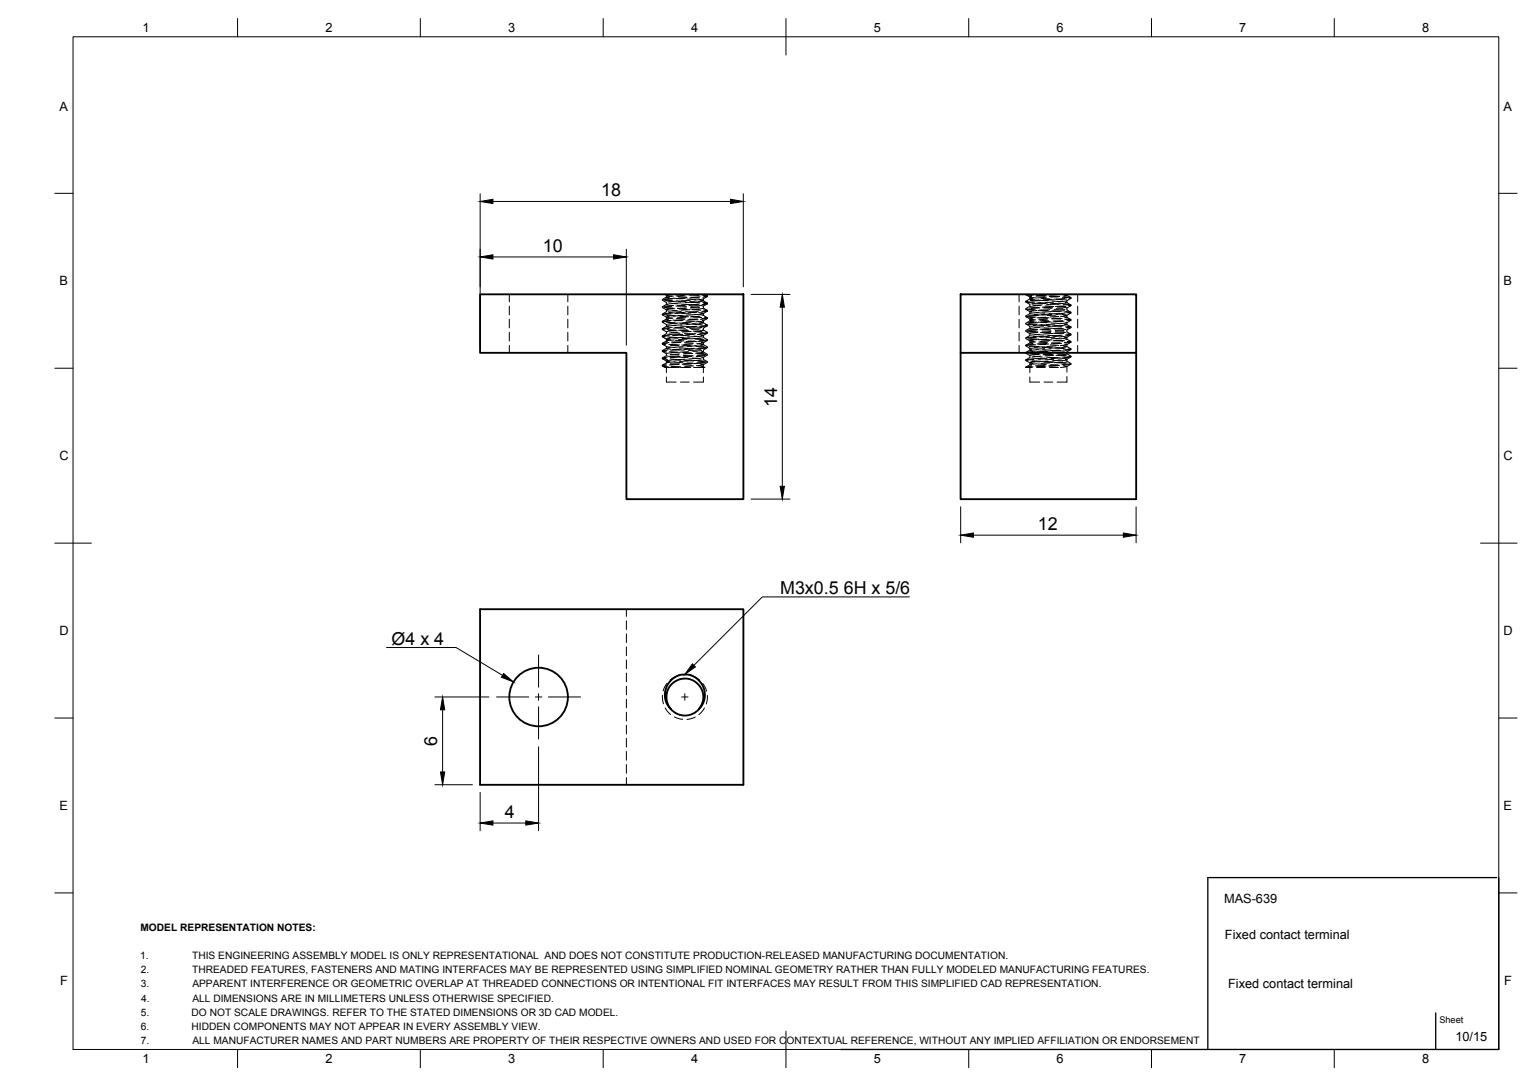
ISO-10303-21;
HEADER;
/* Generated by software containing ST-Developer
 * from STEP Tools, Inc. (www.steptools.com) 
 */

FILE_DESCRIPTION(
/* description */ ('Independent maintained push-to-latch/pull-to-reset mushroom-operator 
CAD. Two opposed spring-loaded ball detents in turned circular seats b
ias both travel stops; direct normally-closed bridge opens6mm when pre
ssed. Rounded palm/pull rim, captured head screw, removable detent clo
sures, native Coil spring families, insulated shared terminals and ord
inary machining features. Manual geometric states and ideal same-mater
ial spring-energy direction only; no electrical/safety certification, 
force/contact dynamics, wear, load or life rating. Requested blue/gray
 visual palette, not safety identification. External wiring/anchors an
d application engineering omitted.'),
/* implementation_level */ '2;1');

FILE_NAME(
/* name */ 'Fixed contact terminal.step',
/* time_stamp */ '2026-11-08T17:54:26-08:00',
/* author */ (''),
/* organization */ (''),
/* preprocessor_version */ 'ST-DEVELOPER v20.2',
/* originating_system */ 'Autodesk Translation Framework v15.17.0.0',
/* authorisation */ '');

FILE_SCHEMA (('AUTOMOTIVE_DESIGN { 1 0 10303 214 3 1 1 }'));
ENDSEC;

DATA;
#10=MECHANICAL_DESIGN_GEOMETRIC_PRESENTATION_REPRESENTATION('',(#198),#43980);
#164=SHAPE_REPRESENTATION_RELATIONSHIP('SRR','None',#44064,#181);
#181=ADVANCED_BREP_SHAPE_REPRESENTATION('',(#215),#43971);
#198=STYLED_ITEM('',(#44154),#215);
#215=MANIFOLD_SOLID_BREP('Body1',#11239);
#247=B_SPLINE_SURFACE_WITH_KNOTS('',3,3,((#35123,#35124,#35125,#35126,#35127,
#35128,#35129,#35130,#35131,#35132,#35133,#35134,#35135,#35136,#35137,#35138,
#35139,#35140,#35141,#35142,#35143,#35144,#35145,#35146,#35147,#35148,#35149,
#35150,#35151,#35152,#35153,#35154,#35155,#35156,#35157,#35158,#35159,#35160,
#35161,#35162,#35163,#35164,#35165,#35166,#35167,#35168,#35169,#35170,#35171,
#35172,#35173,#35174,#35175,#35176,#35177,#35178,#35179,#35180,#35181,#35182,
#35183,#35184,#35185,#35186,#35187,#35188,#35189,#35190),(#35191,#35192,
#35193,#35194,#35195,#35196,#35197,#35198,#35199,#35200,#35201,#35202,#35203,
#35204,#35205,#35206,#35207,#35208,#35209,#35210,#35211,#35212,#35213,#35214,
#35215,#35216,#35217,#35218,#35219,#35220,#35221,#35222,#35223,#35224,#35225,
#35226,#35227,#35228,#35229,#35230,#35231,#35232,#35233,#35234,#35235,#35236,
#35237,#35238,#35239,#35240,#35241,#35242,#35243,#35244,#35245,#35246,#35247,
#35248,#35249,#35250,#35251,#35252,#35253,#35254,#35255,#35256,#35257,#35258),
(#35259,#35260,#35261,#35262,#35263,#35264,#35265,#35266,#35267,#35268,
#35269,#35270,#35271,#35272,#35273,#35274,#35275,#35276,#35277,#35278,#35279,
#35280,#35281,#35282,#35283,#35284,#35285,#35286,#35287,#35288,#35289,#35290,
#35291,#35292,#35293,#35294,#35295,#35296,#35297,#35298,#35299,#35300,#35301,
#35302,#35303,#35304,#35305,#35306,#35307,#35308,#35309,#35310,#35311,#35312,
#35313,#35314,#35315,#35316,#35317,#35318,#35319,#35320,#35321,#35322,#35323,
#35324,#35325,#35326),(#35327,#35328,#35329,#35330,#35331,#35332,#35333,
#35334,#35335,#35336,#35337,#35338,#35339,#35340,#35341,#35342,#35343,#35344,
#35345,#35346,#35347,#35348,#35349,#35350,#35351,#35352,#35353,#35354,#35355,
#35356,#35357,#35358,#35359,#35360,#35361,#35362,#35363,#35364,#35365,#35366,
#35367,#35368,#35369,#35370,#35371,#35372,#35373,#35374,#35375,#35376,#35377,
#35378,#35379,#35380,#35381,#35382,#35383,#35384,#35385,#35386,#35387,#35388,
#35389,#35390,#35391,#35392,#35393,#35394)),.UNSPECIFIED.,.F.,.F.,.F.,(4,
4),(4,1,1,1,1,1,1,1,1,1,1,1,1,1,1,1,1,1,1,1,1,1,1,1,1,1,1,1,1,1,1,1,1,1,
1,1,1,1,1,1,1,1,1,1,1,1,1,1,1,1,1,1,1,1,1,1,1,1,1,1,1,1,1,1,1,4),(0.,0.0321584099938621),
(11.8553612635792,12.8530908876339,13.8508205116886,14.8485501357432,15.8462797597979,
16.8440093838525,17.8417390079072,18.8394686319618,19.8371982560165,20.8349278800712,
21.8326575041258,22.8303871281805,23.8281167522351,24.8258463762898,25.8235760003445,
26.8213056243991,27.8190352484538,28.8167648725084,29.8144944965631,30.8122241206177,
31.8099537446724,32.8076833687271,33.8054129927817,34.8031426168364,35.800872240891,
36.7986018649457,37.7963314890004,38.794061113055,39.7917907371097,40.7895203611643,
41.787249985219,42.7849796092736,43.7827092333283,44.780438857383,45.7781684814376,
46.7758981054923,47.7736277295469,48.7713573536016,49.7690869776563,50.7668166017109,
51.7645462257656,52.7622758498202,53.7600054738749,54.7577350979295,55.7554647219842,
56.7531943460389,57.7509239700935,58.7486535941482,59.7463832182028,60.7441128422575,
61.7418424663121,62.7395720903668,63.7373017144215,64.7350313384761,65.7327609625308,
66.7304905865854,67.7282202106401,68.7259498346948,69.7236794587494,70.7214090828041,
71.7191387068587,72.7168683309134,73.7145979549681,74.7123275790227,75.7100572030774,
76.707786827132),.UNSPECIFIED.);
#248=B_SPLINE_SURFACE_WITH_KNOTS('',3,3,((#35469,#35470,#35471,#35472,#35473,
#35474,#35475,#35476,#35477,#35478,#35479,#35480,#35481,#35482,#35483,#35484,
#35485,#35486,#35487,#35488,#35489,#35490,#35491,#35492,#35493,#35494,#35495,
#35496,#35497,#35498,#35499,#35500,#35501,#35502,#35503,#35504,#35505,#35506,
#35507,#35508,#35509,#35510,#35511,#35512,#35513,#35514,#35515,#35516,#35517,
#35518,#35519,#35520,#35521,#35522,#35523,#35524,#35525,#35526,#35527,#35528,
#35529,#35530,#35531,#35532,#35533,#35534,#35535,#35536),(#35537,#35538,
#35539,#35540,#35541,#35542,#35543,#35544,#35545,#35546,#35547,#35548,#35549,
#35550,#35551,#35552,#35553,#35554,#35555,#35556,#35557,#35558,#35559,#35560,
#35561,#35562,#35563,#35564,#35565,#35566,#35567,#35568,#35569,#35570,#35571,
#35572,#35573,#35574,#35575,#35576,#35577,#35578,#35579,#35580,#35581,#35582,
#35583,#35584,#35585,#35586,#35587,#35588,#35589,#35590,#35591,#35592,#35593,
#35594,#35595,#35596,#35597,#35598,#35599,#35600,#35601,#35602,#35603,#35604),
(#35605,#35606,#35607,#35608,#35609,#35610,#35611,#35612,#35613,#35614,
#35615,#35616,#35617,#35618,#35619,#35620,#35621,#35622,#35623,#35624,#35625,
#35626,#35627,#35628,#35629,#35630,#35631,#35632,#35633,#35634,#35635,#35636,
#35637,#35638,#35639,#35640,#35641,#35642,#35643,#35644,#35645,#35646,#35647,
#35648,#35649,#35650,#35651,#35652,#35653,#35654,#35655,#35656,#35657,#35658,
#35659,#35660,#35661,#35662,#35663,#35664,#35665,#35666,#35667,#35668,#35669,
#35670,#35671,#35672),(#35673,#35674,#35675,#35676,#35677,#35678,#35679,
#35680,#35681,#35682,#35683,#35684,#35685,#35686,#35687,#35688,#35689,#35690,
#35691,#35692,#35693,#35694,#35695,#35696,#35697,#35698,#35699,#35700,#35701,
#35702,#35703,#35704,#35705,#35706,#35707,#35708,#35709,#35710,#35711,#35712,
#35713,#35714,#35715,#35716,#35717,#35718,#35719,#35720,#35721,#35722,#35723,
#35724,#35725,#35726,#35727,#35728,#35729,#35730,#35731,#35732,#35733,#35734,
#35735,#35736,#35737,#35738,#35739,#35740)),.UNSPECIFIED.,.F.,.F.,.F.,(4,
4),(4,1,1,1,1,1,1,1,1,1,1,1,1,1,1,1,1,1,1,1,1,1,1,1,1,1,1,1,1,1,1,1,1,1,
1,1,1,1,1,1,1,1,1,1,1,1,1,1,1,1,1,1,1,1,1,1,1,1,1,1,1,1,1,1,1,4),(0.,0.0321584099938616),
(14.3984001269718,15.3961297510265,16.3938593750811,17.3915889991358,18.3893186231905,
19.3870482472451,20.3847778712998,21.3825074953544,22.3802371194091,23.3779667434637,
24.3756963675184,25.3734259915731,26.3711556156277,27.3688852396824,28.366614863737,
29.3643444877917,30.3620741118463,31.359803735901,32.3575333599556,33.3552629840103,
34.352992608065,35.3507222321196,36.3484518561743,37.3461814802289,38.3439111042836,
39.3416407283382,40.3393703523929,41.3370999764475,42.3348296005022,43.3325592245569,
44.3302888486115,45.3280184726662,46.3257480967208,47.3234777207755,48.3212073448301,
49.3189369688848,50.3166665929395,51.3143962169941,52.3121258410488,53.3098554651034,
54.3075850891581,55.3053147132127,56.3030443372674,57.3007739613221,58.2985035853767,
59.2962332094314,60.293962833486,61.2916924575407,62.2894220815953,63.28715170565,
64.2848813297046,65.2826109537593,66.280340577814,67.2780702018686,68.2757998259233,
69.2735294499779,70.2712590740326,71.2689886980872,72.2667183221419,73.2644479461966,
74.2621775702512,75.2599071943059,76.2576368183605,77.2553664424152,78.2530960664698,
79.2508256905245),.UNSPECIFIED.);
#317=FACE_BOUND('',#1609,.T.);
#318=FACE_BOUND('',#1615,.T.);
#319=FACE_BOUND('',#1616,.T.);
#423=PLANE('',#12010);
#424=PLANE('',#12013);
#425=PLANE('',#12017);
#426=PLANE('',#12018);
#427=PLANE('',#12019);
#428=PLANE('',#12020);
#429=PLANE('',#12021);
#430=PLANE('',#12022);
#431=PLANE('',#12023);
#432=PLANE('',#12024);
#899=FACE_OUTER_BOUND('',#1580,.T.);
#900=FACE_OUTER_BOUND('',#1581,.T.);
#901=FACE_OUTER_BOUND('',#1582,.T.);
#902=FACE_OUTER_BOUND('',#1583,.T.);
#903=FACE_OUTER_BOUND('',#1584,.T.);
#904=FACE_OUTER_BOUND('',#1585,.T.);
#905=FACE_OUTER_BOUND('',#1586,.T.);
#906=FACE_OUTER_BOUND('',#1587,.T.);
#907=FACE_OUTER_BOUND('',#1588,.T.);
#908=FACE_OUTER_BOUND('',#1589,.T.);
#909=FACE_OUTER_BOUND('',#1590,.T.);
#910=FACE_OUTER_BOUND('',#1591,.T.);
#911=FACE_OUTER_BOUND('',#1592,.T.);
#912=FACE_OUTER_BOUND('',#1593,.T.);
#913=FACE_OUTER_BOUND('',#1594,.T.);
#914=FACE_OUTER_BOUND('',#1595,.T.);
#915=FACE_OUTER_BOUND('',#1596,.T.);
#916=FACE_OUTER_BOUND('',#1597,.T.);
#917=FACE_OUTER_BOUND('',#1598,.T.);
#918=FACE_OUTER_BOUND('',#1599,.T.);
#919=FACE_OUTER_BOUND('',#1600,.T.);
#920=FACE_OUTER_BOUND('',#1601,.T.);
#921=FACE_OUTER_BOUND('',#1602,.T.);
#922=FACE_OUTER_BOUND('',#1603,.T.);
#923=FACE_OUTER_BOUND('',#1604,.T.);
#924=FACE_OUTER_BOUND('',#1605,.T.);
#925=FACE_OUTER_BOUND('',#1606,.T.);
#926=FACE_OUTER_BOUND('',#1607,.T.);
#927=FACE_OUTER_BOUND('',#1608,.T.);
#928=FACE_OUTER_BOUND('',#1610,.T.);
#929=FACE_OUTER_BOUND('',#1611,.T.);
#930=FACE_OUTER_BOUND('',#1612,.T.);
#931=FACE_OUTER_BOUND('',#1613,.T.);
#932=FACE_OUTER_BOUND('',#1614,.T.);
#933=FACE_OUTER_BOUND('',#1617,.T.);
#1580=EDGE_LOOP('',(#9101,#9102,#9103,#9104,#9105,#9106,#9107,#9108));
#1581=EDGE_LOOP('',(#9109,#9110,#9111,#9112));
#1582=EDGE_LOOP('',(#9113,#9114,#9115,#9116));
#1583=EDGE_LOOP('',(#9117,#9118,#9119,#9120));
#1584=EDGE_LOOP('',(#9121,#9122,#9123,#9124));
#1585=EDGE_LOOP('',(#9125,#9126,#9127,#9128));
#1586=EDGE_LOOP('',(#9129,#9130,#9131,#9132));
#1587=EDGE_LOOP('',(#9133,#9134,#9135,#9136));
#1588=EDGE_LOOP('',(#9137,#9138,#9139,#9140));
#1589=EDGE_LOOP('',(#9141,#9142,#9143,#9144));
#1590=EDGE_LOOP('',(#9145,#9146,#9147,#9148));
#1591=EDGE_LOOP('',(#9149,#9150,#9151,#9152));
#1592=EDGE_LOOP('',(#9153,#9154,#9155,#9156));
#1593=EDGE_LOOP('',(#9157,#9158,#9159,#9160));
#1594=EDGE_LOOP('',(#9161,#9162,#9163,#9164));
#1595=EDGE_LOOP('',(#9165,#9166,#9167,#9168));
#1596=EDGE_LOOP('',(#9169,#9170,#9171,#9172));
#1597=EDGE_LOOP('',(#9173,#9174,#9175,#9176));
#1598=EDGE_LOOP('',(#9177,#9178,#9179,#9180));
#1599=EDGE_LOOP('',(#9181,#9182,#9183,#9184));
#1600=EDGE_LOOP('',(#9185,#9186,#9187,#9188,#9189));
#1601=EDGE_LOOP('',(#9190,#9191,#9192,#9193));
#1602=EDGE_LOOP('',(#9194,#9195,#9196,#9197,#9198,#9199,#9200,#9201,#9202,
#9203,#9204,#9205,#9206,#9207,#9208,#9209,#9210,#9211,#9212,#9213,#9214,
#9215,#9216,#9217));
#1603=EDGE_LOOP('',(#9218,#9219,#9220,#9221,#9222,#9223,#9224,#9225,#9226,
#9227,#9228,#9229,#9230,#9231,#9232,#9233,#9234,#9235,#9236,#9237,#9238,
#9239,#9240,#9241));
#1604=EDGE_LOOP('',(#9242,#9243,#9244,#9245));
#1605=EDGE_LOOP('',(#9246));
#1606=EDGE_LOOP('',(#9247,#9248,#9249,#9250));
#1607=EDGE_LOOP('',(#9251,#9252,#9253,#9254));
#1608=EDGE_LOOP('',(#9255,#9256,#9257,#9258));
#1609=EDGE_LOOP('',(#9259));
#1610=EDGE_LOOP('',(#9260,#9261,#9262,#9263,#9264,#9265));
#1611=EDGE_LOOP('',(#9266,#9267,#9268,#9269));
#1612=EDGE_LOOP('',(#9270,#9271,#9272,#9273,#9274,#9275));
#1613=EDGE_LOOP('',(#9276,#9277,#9278,#9279));
#1614=EDGE_LOOP('',(#9280,#9281,#9282,#9283));
#1615=EDGE_LOOP('',(#9284,#9285,#9286,#9287));
#1616=EDGE_LOOP('',(#9288));
#1617=EDGE_LOOP('',(#9289,#9290,#9291,#9292));
#1947=CIRCLE('',#11985,0.12645);
#1948=CIRCLE('',#11986,0.12645);
#1949=CIRCLE('',#11987,0.12645);
#1950=CIRCLE('',#11997,0.12645);
#1951=CIRCLE('',#11999,0.1543);
#1952=CIRCLE('',#12009,0.1543);
#1953=CIRCLE('',#12015,0.2);
#1954=CIRCLE('',#12016,0.2);
#2561=B_SPLINE_CURVE_WITH_KNOTS('',3,(#34297,#34298,#34299,#34300),
 .UNSPECIFIED.,.F.,.F.,(4,4),(64.1414162127729,64.8524255635527),
 .UNSPECIFIED.);
#2562=B_SPLINE_CURVE_WITH_KNOTS('',3,(#34308,#34309,#34310,#34311,#34312,
#34313,#34314,#34315,#34316,#34317),.UNSPECIFIED.,.F.,.F.,(4,3,3,4),(-62.8318530717959,
-61.8592366913888,-60.8615070673342,-60.401269768986),.UNSPECIFIED.);
#2563=B_SPLINE_CURVE_WITH_KNOTS('',3,(#34322,#34323,#34324,#34325,#34326,
#34327,#34328,#34329,#34330,#34331,#34332,#34333,#34334,#34335,#34336,#34337,
#34338,#34339,#34340,#34341,#34342,#34343,#34344,#34345,#34346),
 .UNSPECIFIED.,.F.,.F.,(4,3,3,3,3,3,3,3,4),(57.8582309055934,57.8683181951701,
58.8660478192247,59.8637774432794,60.861507067334,61.8592366913887,62.8569663154434,
63.854695939498,64.1414162127729),.UNSPECIFIED.);
#2564=B_SPLINE_CURVE_WITH_KNOTS('',3,(#34347,#34348,#34349,#34350,#34351,
#34352,#34353,#34354,#34355,#34356,#34357,#34358,#34359,#34360,#34361,#34362,
#34363,#34364,#34365,#34366,#34367,#34368),.UNSPECIFIED.,.F.,.F.,(4,3,3,
3,3,3,3,4),(-60.401269768986,-59.8637774432795,-58.8660478192248,-57.8683181951702,
-56.8705885711155,-55.8728589470609,-54.8751293230062,-54.1180844618064),
 .UNSPECIFIED.);
#2565=B_SPLINE_CURVE_WITH_KNOTS('',3,(#34373,#34374,#34375,#34376,#34377,
#34378,#34379,#34380,#34381,#34382,#34383,#34384,#34385,#34386,#34387,#34388,
#34389,#34390,#34391,#34392,#34393,#34394),.UNSPECIFIED.,.F.,.F.,(4,3,3,
3,3,3,3,4),(51.5750455984138,51.8819404508421,52.8796700748968,53.8773996989514,
54.8751293230061,55.8728589470608,56.8705885711154,57.8582309055934),
 .UNSPECIFIED.);
#2566=B_SPLINE_CURVE_WITH_KNOTS('',3,(#34395,#34396,#34397,#34398,#34399,
#34400,#34401,#34402,#34403,#34404,#34405,#34406,#34407,#34408,#34409,#34410,
#34411,#34412,#34413,#34414,#34415,#34416,#34417,#34418,#34419),
 .UNSPECIFIED.,.F.,.F.,(4,3,3,3,3,3,3,3,4),(-54.1180844618064,-53.8773996989516,
-52.8796700748969,-51.8819404508422,-50.8842108267876,-49.8864812027329,
-48.8887515786783,-47.8910219546236,-47.8348991546268),.UNSPECIFIED.);
#2567=B_SPLINE_CURVE_WITH_KNOTS('',3,(#34424,#34425,#34426,#34427,#34428,
#34429,#34430,#34431,#34432,#34433,#34434,#34435,#34436,#34437,#34438,#34439,
#34440,#34441,#34442,#34443,#34444,#34445),.UNSPECIFIED.,.F.,.F.,(4,3,3,
3,3,3,3,4),(45.2918602912342,45.8955627065142,46.8932923305688,47.8910219546235,
48.8887515786782,49.8864812027328,50.8842108267875,51.5750455984138),
 .UNSPECIFIED.);
#2568=B_SPLINE_CURVE_WITH_KNOTS('',3,(#34446,#34447,#34448,#34449,#34450,
#34451,#34452,#34453,#34454,#34455,#34456,#34457,#34458,#34459,#34460,#34461,
#34462,#34463,#34464,#34465,#34466,#34467),.UNSPECIFIED.,.F.,.F.,(4,3,3,
3,3,3,3,4),(-47.8348991546268,-46.8932923305689,-45.8955627065143,-44.8978330824596,
-43.900103458405,-42.9023738343503,-41.9046442102957,-41.5517138474472),
 .UNSPECIFIED.);
#2569=B_SPLINE_CURVE_WITH_KNOTS('',3,(#34472,#34473,#34474,#34475,#34476,
#34477,#34478,#34479,#34480,#34481,#34482,#34483,#34484,#34485,#34486,#34487,
#34488,#34489,#34490,#34491,#34492,#34493),.UNSPECIFIED.,.F.,.F.,(4,3,3,
3,3,3,3,4),(39.0086749840546,39.9091849621863,40.9069145862409,41.9046442102956,
42.9023738343502,43.9001034584049,44.8978330824595,45.2918602912342),
 .UNSPECIFIED.);
#2570=B_SPLINE_CURVE_WITH_KNOTS('',3,(#34494,#34495,#34496,#34497,#34498,
#34499,#34500,#34501,#34502,#34503,#34504,#34505,#34506,#34507,#34508,#34509,
#34510,#34511,#34512,#34513,#34514,#34515),.UNSPECIFIED.,.F.,.F.,(4,3,3,
3,3,3,3,4),(-41.5517138474472,-40.906914586241,-39.9091849621863,-38.9114553381317,
-37.913725714077,-36.9159960900224,-35.9182664659677,-35.2685285402676),
 .UNSPECIFIED.);
#2571=B_SPLINE_CURVE_WITH_KNOTS('',3,(#34520,#34521,#34522,#34523,#34524,
#34525,#34526,#34527,#34528,#34529,#34530,#34531,#34532,#34533,#34534,#34535,
#34536,#34537,#34538,#34539,#34540,#34541,#34542,#34543,#34544),
 .UNSPECIFIED.,.F.,.F.,(4,3,3,3,3,3,3,3,4),(32.725489676875,32.9250775938037,
33.9228072178583,34.920536841913,35.9182664659676,36.9159960900223,37.9137257140769,
38.9114553381316,39.0086749840546),.UNSPECIFIED.);
#2572=B_SPLINE_CURVE_WITH_KNOTS('',3,(#34545,#34546,#34547,#34548,#34549,
#34550,#34551,#34552,#34553,#34554,#34555,#34556,#34557,#34558,#34559,#34560,
#34561,#34562,#34563,#34564,#34565,#34566),.UNSPECIFIED.,.F.,.F.,(4,3,3,
3,3,3,3,4),(-35.2685285402676,-34.920536841913,-33.9228072178584,-32.9250775938037,
-31.9273479697491,-30.9296183456944,-29.9318887216397,-28.985343233088),
 .UNSPECIFIED.);
#2573=B_SPLINE_CURVE_WITH_KNOTS('',3,(#34571,#34572,#34573,#34574,#34575,
#34576,#34577,#34578,#34579,#34580,#34581,#34582,#34583,#34584,#34585,#34586,
#34587,#34588,#34589,#34590,#34591,#34592),.UNSPECIFIED.,.F.,.F.,(4,3,3,
3,3,3,3,4),(26.4423043696954,26.9386998494757,27.9364294735304,28.934159097585,
29.9318887216397,30.9296183456943,31.927347969749,32.725489676875),
 .UNSPECIFIED.);
#2574=B_SPLINE_CURVE_WITH_KNOTS('',3,(#34593,#34594,#34595,#34596,#34597,
#34598,#34599,#34600,#34601,#34602,#34603,#34604,#34605,#34606,#34607,#34608,
#34609,#34610,#34611,#34612,#34613,#34614,#34615,#34616,#34617),
 .UNSPECIFIED.,.F.,.F.,(4,3,3,3,3,3,3,3,4),(-28.985343233088,-28.9341590975851,
-27.9364294735304,-26.9386998494758,-25.9409702254211,-24.9432406013665,
-23.9455109773118,-22.9477813532571,-22.7021579259084),.UNSPECIFIED.);
#2575=B_SPLINE_CURVE_WITH_KNOTS('',3,(#34622,#34623,#34624,#34625,#34626,
#34627,#34628,#34629,#34630,#34631,#34632,#34633,#34634,#34635,#34636,#34637,
#34638,#34639,#34640,#34641,#34642,#34643),.UNSPECIFIED.,.F.,.F.,(4,3,3,
3,3,3,3,4),(20.1591190625158,20.9523221051478,21.9500517292024,22.9477813532571,
23.9455109773117,24.9432406013664,25.9409702254211,26.4423043696954),
 .UNSPECIFIED.);
#2576=B_SPLINE_CURVE_WITH_KNOTS('',3,(#34644,#34645,#34646,#34647,#34648,
#34649,#34650,#34651,#34652,#34653,#34654,#34655,#34656,#34657,#34658,#34659,
#34660,#34661,#34662,#34663,#34664,#34665),.UNSPECIFIED.,.F.,.F.,(4,3,3,
3,3,3,3,4),(-22.7021579259084,-21.9500517292025,-20.9523221051478,-19.9545924810932,
-18.9568628570385,-17.9591332329838,-16.9614036089292,-16.4189726187288),
 .UNSPECIFIED.);
#2577=B_SPLINE_CURVE_WITH_KNOTS('',3,(#34670,#34671,#34672,#34673,#34674,
#34675,#34676,#34677,#34678,#34679,#34680,#34681,#34682,#34683,#34684,#34685,
#34686,#34687,#34688,#34689,#34690,#34691,#34692,#34693,#34694),
 .UNSPECIFIED.,.F.,.F.,(4,3,3,3,3,3,3,3,4),(13.8759337553362,13.9682147367652,
14.9659443608198,15.9636739848745,16.9614036089292,17.9591332329838,18.9568628570385,
19.9545924810931,20.1591190625158),.UNSPECIFIED.);
#2578=B_SPLINE_CURVE_WITH_KNOTS('',3,(#34695,#34696,#34697,#34698,#34699,
#34700,#34701,#34702,#34703,#34704,#34705,#34706,#34707,#34708,#34709,#34710,
#34711,#34712,#34713,#34714,#34715,#34716),.UNSPECIFIED.,.F.,.F.,(4,3,3,
3,3,3,3,4),(-16.4189726187288,-15.9636739848745,-14.9659443608199,-13.9682147367652,
-12.9704851127106,-11.9727554886559,-10.9750258646012,-10.1357873115493),
 .UNSPECIFIED.);
#2579=B_SPLINE_CURVE_WITH_KNOTS('',3,(#34722,#34723,#34724,#34725,#34726,
#34727,#34728,#34729,#34730,#34731,#34732,#34733,#34734),.UNSPECIFIED.,
 .F.,.F.,(4,3,3,3,4),(-3.85260200436966,-2.99318887216398,-1.99545924810932,
-0.997729624054659,0.),.UNSPECIFIED.);
#2580=B_SPLINE_CURVE_WITH_KNOTS('',3,(#34737,#34738,#34739,#34740,#34741,
#34742,#34743,#34744,#34745,#34746,#34747,#34748,#34749,#34750,#34751,#34752,
#34753,#34754,#34755),.UNSPECIFIED.,.F.,.F.,(4,3,3,3,3,3,4),(2.02057249175679,
2.99318887216397,3.99091849621862,4.98864812027328,5.98637774432793,6.98410736838259,
7.59274844815664),.UNSPECIFIED.);
#2581=B_SPLINE_CURVE_WITH_KNOTS('',3,(#34761,#34762,#34763,#34764,#34765,
#34766,#34767,#34768),.UNSPECIFIED.,.F.,.F.,(4,1,1,1,1,4),(72.2566310325653,
72.7168683309134,73.7145979549681,74.7123275790227,75.7100572030774,76.707786827132),
 .UNSPECIFIED.);
#2582=B_SPLINE_CURVE_WITH_KNOTS('',3,(#34771,#34772,#34773,#34774,#34775,
#34776,#34777,#34778,#34779),.UNSPECIFIED.,.F.,.F.,(4,1,1,1,1,1,4),(72.2566310325653,
72.2667183221419,73.2644479461966,74.2621775702512,75.2599071943059,76.2576368183605,
77.2302531987677),.UNSPECIFIED.);
#2583=B_SPLINE_CURVE_WITH_KNOTS('',3,(#34784,#34785,#34786,#34787,#34788,
#34789,#34790,#34791,#34792,#34793),.UNSPECIFIED.,.F.,.F.,(4,1,1,1,1,1,
1,4),(65.9734457253856,66.7304905865854,67.7282202106401,68.7259498346948,
69.7236794587494,70.7214090828041,71.7191387068587,72.2566310325653),
 .UNSPECIFIED.);
#2584=B_SPLINE_CURVE_WITH_KNOTS('',3,(#34794,#34795,#34796,#34797,#34798,
#34799,#34800,#34801,#34802,#34803),.UNSPECIFIED.,.F.,.F.,(4,1,1,1,1,1,
1,4),(65.9734457253856,66.280340577814,67.2780702018686,68.2757998259233,
69.2735294499779,70.2712590740326,71.2689886980872,72.2566310325653),
 .UNSPECIFIED.);
#2585=B_SPLINE_CURVE_WITH_KNOTS('',3,(#34808,#34809,#34810,#34811,#34812,
#34813,#34814,#34815,#34816,#34817,#34818),.UNSPECIFIED.,.F.,.F.,(4,1,1,
1,1,1,1,1,4),(59.690260418206,59.7463832182028,60.7441128422575,61.7418424663121,
62.7395720903668,63.7373017144215,64.7350313384761,65.7327609625308,65.9734457253856),
 .UNSPECIFIED.);
#2586=B_SPLINE_CURVE_WITH_KNOTS('',3,(#34819,#34820,#34821,#34822,#34823,
#34824,#34825,#34826,#34827,#34828),.UNSPECIFIED.,.F.,.F.,(4,1,1,1,1,1,
1,4),(59.690260418206,60.293962833486,61.2916924575407,62.2894220815953,
63.28715170565,64.2848813297046,65.2826109537593,65.9734457253856),
 .UNSPECIFIED.);
#2587=B_SPLINE_CURVE_WITH_KNOTS('',3,(#34833,#34834,#34835,#34836,#34837,
#34838,#34839,#34840,#34841,#34842),.UNSPECIFIED.,.F.,.F.,(4,1,1,1,1,1,
1,4),(53.4070751110265,53.7600054738749,54.7577350979295,55.7554647219842,
56.7531943460389,57.7509239700935,58.7486535941482,59.690260418206),
 .UNSPECIFIED.);
#2588=B_SPLINE_CURVE_WITH_KNOTS('',3,(#34843,#34844,#34845,#34846,#34847,
#34848,#34849,#34850,#34851,#34852),.UNSPECIFIED.,.F.,.F.,(4,1,1,1,1,1,
1,4),(53.4070751110265,54.3075850891581,55.3053147132127,56.3030443372674,
57.3007739613221,58.2985035853767,59.2962332094314,59.690260418206),
 .UNSPECIFIED.);
#2589=B_SPLINE_CURVE_WITH_KNOTS('',3,(#34857,#34858,#34859,#34860,#34861,
#34862,#34863,#34864,#34865,#34866),.UNSPECIFIED.,.F.,.F.,(4,1,1,1,1,1,
1,4),(47.1238898038468,47.7736277295469,48.7713573536016,49.7690869776563,
50.7668166017109,51.7645462257656,52.7622758498202,53.4070751110265),
 .UNSPECIFIED.);
#2590=B_SPLINE_CURVE_WITH_KNOTS('',3,(#34867,#34868,#34869,#34870,#34871,
#34872,#34873,#34874,#34875,#34876,#34877),.UNSPECIFIED.,.F.,.F.,(4,1,1,
1,1,1,1,1,4),(47.1238898038468,47.3234777207755,48.3212073448301,49.3189369688848,
50.3166665929395,51.3143962169941,52.3121258410488,53.3098554651034,53.4070751110265),
 .UNSPECIFIED.);
#2591=B_SPLINE_CURVE_WITH_KNOTS('',3,(#34882,#34883,#34884,#34885,#34886,
#34887,#34888,#34889,#34890,#34891),.UNSPECIFIED.,.F.,.F.,(4,1,1,1,1,1,
1,4),(40.8407044966673,41.787249985219,42.7849796092736,43.7827092333283,
44.780438857383,45.7781684814376,46.7758981054923,47.1238898038468),
 .UNSPECIFIED.);
#2592=B_SPLINE_CURVE_WITH_KNOTS('',3,(#34892,#34893,#34894,#34895,#34896,
#34897,#34898,#34899,#34900,#34901),.UNSPECIFIED.,.F.,.F.,(4,1,1,1,1,1,
1,4),(40.8407044966673,41.3370999764475,42.3348296005022,43.3325592245569,
44.3302888486115,45.3280184726662,46.3257480967208,47.1238898038468),
 .UNSPECIFIED.);
#2593=B_SPLINE_CURVE_WITH_KNOTS('',3,(#34906,#34907,#34908,#34909,#34910,
#34911,#34912,#34913,#34914,#34915,#34916),.UNSPECIFIED.,.F.,.F.,(4,1,1,
1,1,1,1,1,4),(34.5575191894877,34.8031426168364,35.800872240891,36.7986018649457,
37.7963314890004,38.794061113055,39.7917907371097,40.7895203611643,40.8407044966673),
 .UNSPECIFIED.);
#2594=B_SPLINE_CURVE_WITH_KNOTS('',3,(#34917,#34918,#34919,#34920,#34921,
#34922,#34923,#34924,#34925,#34926),.UNSPECIFIED.,.F.,.F.,(4,1,1,1,1,1,
1,4),(34.5575191894877,35.3507222321196,36.3484518561743,37.3461814802289,
38.3439111042836,39.3416407283382,40.3393703523929,40.8407044966673),
 .UNSPECIFIED.);
#2595=B_SPLINE_CURVE_WITH_KNOTS('',3,(#34931,#34932,#34933,#34934,#34935,
#34936,#34937,#34938,#34939,#34940),.UNSPECIFIED.,.F.,.F.,(4,1,1,1,1,1,
1,4),(28.2743338823081,28.8167648725084,29.8144944965631,30.8122241206177,
31.8099537446724,32.8076833687271,33.8054129927817,34.5575191894877),
 .UNSPECIFIED.);
#2596=B_SPLINE_CURVE_WITH_KNOTS('',3,(#34941,#34942,#34943,#34944,#34945,
#34946,#34947,#34948,#34949,#34950,#34951),.UNSPECIFIED.,.F.,.F.,(4,1,1,
1,1,1,1,1,4),(28.2743338823081,28.366614863737,29.3643444877917,30.3620741118463,
31.359803735901,32.3575333599556,33.3552629840103,34.352992608065,34.5575191894877),
 .UNSPECIFIED.);
#2597=B_SPLINE_CURVE_WITH_KNOTS('',3,(#34956,#34957,#34958,#34959,#34960,
#34961,#34962,#34963,#34964,#34965),.UNSPECIFIED.,.F.,.F.,(4,1,1,1,1,1,
1,4),(21.9911485751285,22.8303871281805,23.8281167522351,24.8258463762898,
25.8235760003445,26.8213056243991,27.8190352484538,28.2743338823081),
 .UNSPECIFIED.);
#2598=B_SPLINE_CURVE_WITH_KNOTS('',3,(#34966,#34967,#34968,#34969,#34970,
#34971,#34972,#34973,#34974,#34975),.UNSPECIFIED.,.F.,.F.,(4,1,1,1,1,1,
1,4),(21.9911485751285,22.3802371194091,23.3779667434637,24.3756963675184,
25.3734259915731,26.3711556156277,27.3688852396824,28.2743338823081),
 .UNSPECIFIED.);
#2599=B_SPLINE_CURVE_WITH_KNOTS('',3,(#34981,#34982,#34983,#34984,#34985),
 .UNSPECIFIED.,.F.,.F.,(4,1,4),(14.3984001269718,15.3961297510265,15.7079632679489),
 .UNSPECIFIED.);
#2600=B_SPLINE_CURVE_WITH_KNOTS('',3,(#34988,#34989,#34990,#34991,#34992),
 .UNSPECIFIED.,.F.,.F.,(4,1,4),(13.8759337553361,14.8485501357432,15.7079632679489),
 .UNSPECIFIED.);
#2601=B_SPLINE_CURVE_WITH_KNOTS('',3,(#34994,#34995,#34996,#34997,#34998,
#34999,#35000,#35001,#35002,#35003,#35004,#35005,#35006,#35007,#35008,#35009,
#35010,#35011,#35012,#35013,#35014,#35015,#35016,#35017,#35018,#35019,#35020,
#35021,#35022,#35023,#35024,#35025,#35026,#35027,#35028,#35029,#35030,#35031,
#35032,#35033,#35034,#35035,#35036,#35037,#35038,#35039,#35040,#35041,#35042,
#35043,#35044,#35045),.UNSPECIFIED.,.F.,.F.,(4,3,3,3,3,3,3,3,3,3,3,3,3,
3,3,3,3,4),(-0.286347380332243,-0.266225517657927,-0.253989633145399,-0.224118418951897,
-0.213637228539926,-0.18277997814213,-0.1712802294816,-0.161583702204544,
-0.151922727744335,-0.129977880386141,-0.117970426661857,-0.109303558462843,
-0.0829498108000933,-0.0663205445941391,-0.0521986510922473,-0.0198616494821571,
-0.00388856781184301,0.),.UNSPECIFIED.);
#2602=B_SPLINE_CURVE_WITH_KNOTS('',3,(#35046,#35047,#35048,#35049,#35050,
#35051,#35052,#35053,#35054,#35055,#35056,#35057,#35058,#35059,#35060,#35061,
#35062,#35063,#35064,#35065,#35066,#35067,#35068,#35069,#35070,#35071,#35072,
#35073,#35074,#35075,#35076,#35077,#35078,#35079,#35080,#35081,#35082,#35083,
#35084,#35085,#35086,#35087,#35088,#35089,#35090,#35091,#35092,#35093,#35094,
#35095,#35096,#35097,#35098,#35099,#35100),.UNSPECIFIED.,.F.,.F.,(4,3,3,
3,3,3,3,3,3,3,3,3,3,3,3,3,3,3,4),(-0.285142803995136,-0.264771978453909,
-0.248971203111392,-0.236527824899921,-0.214293390992849,-0.2038268270722,
-0.17295400685889,-0.159192875564253,-0.149652609754856,-0.137562774558619,
-0.11631964633286,-0.104925727456541,-0.0956925453293139,-0.0725695145406395,
-0.0586514835868502,-0.0490375298028169,-0.0212486353032901,-0.00320042217461625,
0.),.UNSPECIFIED.);
#2603=B_SPLINE_CURVE_WITH_KNOTS('',3,(#35102,#35103,#35104,#35105,#35106,
#35107,#35108,#35109,#35110,#35111,#35112),.UNSPECIFIED.,.F.,.F.,(4,1,1,
1,1,1,1,1,4),(15.7079632679489,15.8462797597979,16.8440093838525,17.8417390079072,
18.8394686319618,19.8371982560165,20.8349278800712,21.8326575041258,21.9911485751285),
 .UNSPECIFIED.);
#2604=B_SPLINE_CURVE_WITH_KNOTS('',3,(#35113,#35114,#35115,#35116,#35117,
#35118,#35119,#35120,#35121,#35122),.UNSPECIFIED.,.F.,.F.,(4,1,1,1,1,1,
1,4),(15.7079632679489,16.3938593750811,17.3915889991358,18.3893186231905,
19.3870482472451,20.3847778712998,21.3825074953544,21.9911485751285),
 .UNSPECIFIED.);
#2605=B_SPLINE_CURVE_WITH_KNOTS('',3,(#35395,#35396,#35397,#35398,#35399,
#35400,#35401,#35402,#35403,#35404,#35405,#35406,#35407,#35408,#35409,#35410,
#35411,#35412,#35413,#35414,#35415,#35416,#35417,#35418,#35419,#35420,#35421,
#35422,#35423,#35424,#35425,#35426,#35427,#35428,#35429,#35430,#35431,#35432,
#35433,#35434,#35435,#35436,#35437,#35438,#35439,#35440,#35441,#35442,#35443),
 .UNSPECIFIED.,.F.,.F.,(4,3,3,3,3,3,3,3,3,3,3,3,3,3,3,3,4),(0.,0.0274255371814078,
0.0484189866654049,0.0576777559231281,0.0872193790463039,0.100313119697051,
0.108749799500732,0.134012411342703,0.149997937188314,0.163168454336766,
0.192693763100972,0.210037636696566,0.220559059471184,0.247872294074534,
0.26049857837061,0.281269689393589,0.285142803995142),.UNSPECIFIED.);
#2606=B_SPLINE_CURVE_WITH_KNOTS('',3,(#35444,#35445,#35446,#35447,#35448,
#35449,#35450,#35451,#35452,#35453,#35454,#35455,#35456,#35457,#35458,#35459,
#35460,#35461,#35462,#35463,#35464,#35465,#35466,#35467,#35468),
 .UNSPECIFIED.,.F.,.F.,(4,3,3,3,3,3,3,3,4),(-10.1357873115493,-9.97729624054658,
-8.97956661649192,-7.98183699243727,-6.98410736838261,-5.98637774432795,
-4.98864812027329,-3.99091849621863,-3.85260200436966),.UNSPECIFIED.);
#2607=B_SPLINE_CURVE_WITH_KNOTS('',3,(#35741,#35742,#35743,#35744,#35745,
#35746,#35747,#35748,#35749,#35750,#35751,#35752,#35753,#35754,#35755,#35756,
#35757,#35758,#35759,#35760,#35761,#35762),.UNSPECIFIED.,.F.,.F.,(4,3,3,
3,3,3,3,4),(7.59274844815664,7.98183699243725,8.9795666164919,9.97729624054656,
10.9750258646012,11.9727554886559,12.9704851127105,13.8759337553362),
 .UNSPECIFIED.);
#2608=B_SPLINE_CURVE_WITH_KNOTS('',3,(#35763,#35764,#35765,#35766,#35767,
#35768,#35769,#35770,#35771,#35772,#35773,#35774,#35775,#35776,#35777,#35778,
#35779,#35780,#35781,#35782,#35783,#35784,#35785,#35786,#35787,#35788,#35789,
#35790,#35791,#35792,#35793,#35794,#35795,#35796,#35797,#35798,#35799,#35800,
#35801,#35802,#35803,#35804,#35805,#35806,#35807,#35808,#35809,#35810,#35811),
 .UNSPECIFIED.,.F.,.F.,(4,3,3,3,3,3,3,3,3,3,3,3,3,3,3,3,4),(0.,0.0320358644790656,
0.0566025392350713,0.0661929095230273,0.097524509655756,0.113218578765797,
0.122777613428698,0.148357330195644,0.170686258066526,0.180239221440332,
0.205963417559621,0.220473935588774,0.231002296372473,0.247562418687567,
0.263621625608468,0.283136005917488,0.286347380332233),.UNSPECIFIED.);
#3235=LINE('',#34295,#3867);
#3236=LINE('',#34304,#3868);
#3237=LINE('',#34321,#3869);
#3238=LINE('',#34372,#3870);
#3239=LINE('',#34423,#3871);
#3240=LINE('',#34471,#3872);
#3241=LINE('',#34519,#3873);
#3242=LINE('',#34570,#3874);
#3243=LINE('',#34621,#3875);
#3244=LINE('',#34669,#3876);
#3245=LINE('',#34720,#3877);
#3246=LINE('',#34759,#3878);
#3247=LINE('',#34783,#3879);
#3248=LINE('',#34807,#3880);
#3249=LINE('',#34832,#3881);
#3250=LINE('',#34856,#3882);
#3251=LINE('',#34881,#3883);
#3252=LINE('',#34905,#3884);
#3253=LINE('',#34930,#3885);
#3254=LINE('',#34955,#3886);
#3255=LINE('',#34979,#3887);
#3256=LINE('',#35818,#3888);
#3257=LINE('',#35823,#3889);
#3258=LINE('',#35825,#3890);
#3259=LINE('',#35827,#3891);
#3260=LINE('',#35828,#3892);
#3261=LINE('',#35832,#3893);
#3262=LINE('',#35833,#3894);
#3263=LINE('',#35834,#3895);
#3264=LINE('',#35837,#3896);
#3265=LINE('',#35839,#3897);
#3266=LINE('',#35841,#3898);
#3267=LINE('',#35842,#3899);
#3268=LINE('',#35845,#3900);
#3269=LINE('',#35846,#3901);
#3270=LINE('',#35849,#3902);
#3271=LINE('',#35851,#3903);
#3272=LINE('',#35852,#3904);
#3273=LINE('',#35854,#3905);
#3274=LINE('',#35855,#3906);
#3867=VECTOR('',#13770,0.15);
#3868=VECTOR('',#13773,0.15);
#3869=VECTOR('',#13780,0.15);
#3870=VECTOR('',#13783,0.15);
#3871=VECTOR('',#13786,0.15);
#3872=VECTOR('',#13789,0.15);
#3873=VECTOR('',#13792,0.15);
#3874=VECTOR('',#13795,0.15);
#3875=VECTOR('',#13798,0.15);
#3876=VECTOR('',#13801,0.15);
#3877=VECTOR('',#13804,0.15);
#3878=VECTOR('',#13809,0.1543);
#3879=VECTOR('',#13814,0.1543);
#3880=VECTOR('',#13817,0.1543);
#3881=VECTOR('',#13820,0.1543);
#3882=VECTOR('',#13823,0.1543);
#3883=VECTOR('',#13826,0.1543);
#3884=VECTOR('',#13829,0.1543);
#3885=VECTOR('',#13832,0.1543);
#3886=VECTOR('',#13835,0.1543);
#3887=VECTOR('',#13838,0.1543);
#3888=VECTOR('',#13853,0.2);
#3889=VECTOR('',#13858,1.);
#3890=VECTOR('',#13859,1.);
#3891=VECTOR('',#13860,1.);
#3892=VECTOR('',#13861,1.);
#3893=VECTOR('',#13864,1.);
#3894=VECTOR('',#13865,1.);
#3895=VECTOR('',#13866,1.);
#3896=VECTOR('',#13869,1.);
#3897=VECTOR('',#13870,1.);
#3898=VECTOR('',#13871,1.);
#3899=VECTOR('',#13872,1.);
#3900=VECTOR('',#13875,1.);
#3901=VECTOR('',#13876,1.);
#3902=VECTOR('',#13879,1.);
#3903=VECTOR('',#13880,1.);
#3904=VECTOR('',#13881,1.);
#3905=VECTOR('',#13884,1.);
#3906=VECTOR('',#13885,1.);
#4838=VERTEX_POINT('',#34293);
#4839=VERTEX_POINT('',#34294);
#4840=VERTEX_POINT('',#34296);
#4841=VERTEX_POINT('',#34301);
#4842=VERTEX_POINT('',#34303);
#4843=VERTEX_POINT('',#34306);
#4844=VERTEX_POINT('',#34319);
#4845=VERTEX_POINT('',#34320);
#4846=VERTEX_POINT('',#34370);
#4847=VERTEX_POINT('',#34371);
#4848=VERTEX_POINT('',#34421);
#4849=VERTEX_POINT('',#34422);
#4850=VERTEX_POINT('',#34469);
#4851=VERTEX_POINT('',#34470);
#4852=VERTEX_POINT('',#34517);
#4853=VERTEX_POINT('',#34518);
#4854=VERTEX_POINT('',#34568);
#4855=VERTEX_POINT('',#34569);
#4856=VERTEX_POINT('',#34619);
#4857=VERTEX_POINT('',#34620);
#4858=VERTEX_POINT('',#34667);
#4859=VERTEX_POINT('',#34668);
#4860=VERTEX_POINT('',#34718);
#4861=VERTEX_POINT('',#34719);
#4862=VERTEX_POINT('',#34721);
#4863=VERTEX_POINT('',#34735);
#4864=VERTEX_POINT('',#34757);
#4865=VERTEX_POINT('',#34758);
#4866=VERTEX_POINT('',#34760);
#4867=VERTEX_POINT('',#34769);
#4868=VERTEX_POINT('',#34781);
#4869=VERTEX_POINT('',#34782);
#4870=VERTEX_POINT('',#34805);
#4871=VERTEX_POINT('',#34806);
#4872=VERTEX_POINT('',#34830);
#4873=VERTEX_POINT('',#34831);
#4874=VERTEX_POINT('',#34854);
#4875=VERTEX_POINT('',#34855);
#4876=VERTEX_POINT('',#34879);
#4877=VERTEX_POINT('',#34880);
#4878=VERTEX_POINT('',#34903);
#4879=VERTEX_POINT('',#34904);
#4880=VERTEX_POINT('',#34928);
#4881=VERTEX_POINT('',#34929);
#4882=VERTEX_POINT('',#34953);
#4883=VERTEX_POINT('',#34954);
#4884=VERTEX_POINT('',#34977);
#4885=VERTEX_POINT('',#34978);
#4886=VERTEX_POINT('',#34980);
#4887=VERTEX_POINT('',#34986);
#4888=VERTEX_POINT('',#35815);
#4889=VERTEX_POINT('',#35817);
#4890=VERTEX_POINT('',#35821);
#4891=VERTEX_POINT('',#35822);
#4892=VERTEX_POINT('',#35824);
#4893=VERTEX_POINT('',#35826);
#4894=VERTEX_POINT('',#35830);
#4895=VERTEX_POINT('',#35831);
#4896=VERTEX_POINT('',#35836);
#4897=VERTEX_POINT('',#35838);
#4898=VERTEX_POINT('',#35840);
#4899=VERTEX_POINT('',#35844);
#4900=VERTEX_POINT('',#35848);
#4901=VERTEX_POINT('',#35850);
#6320=EDGE_CURVE('',#4838,#4839,#3235,.T.);
#6321=EDGE_CURVE('',#4839,#4840,#2561,.T.);
#6322=EDGE_CURVE('',#4840,#4841,#1947,.T.);
#6323=EDGE_CURVE('',#4841,#4842,#3236,.T.);
#6324=EDGE_CURVE('',#4842,#4842,#1948,.F.);
#6325=EDGE_CURVE('',#4841,#4843,#1949,.T.);
#6326=EDGE_CURVE('',#4843,#4838,#2562,.T.);
#6327=EDGE_CURVE('',#4844,#4845,#3237,.T.);
#6328=EDGE_CURVE('',#4845,#4839,#2563,.T.);
#6329=EDGE_CURVE('',#4838,#4844,#2564,.T.);
#6330=EDGE_CURVE('',#4846,#4847,#3238,.T.);
#6331=EDGE_CURVE('',#4847,#4845,#2565,.T.);
#6332=EDGE_CURVE('',#4844,#4846,#2566,.T.);
#6333=EDGE_CURVE('',#4848,#4849,#3239,.T.);
#6334=EDGE_CURVE('',#4849,#4847,#2567,.T.);
#6335=EDGE_CURVE('',#4846,#4848,#2568,.T.);
#6336=EDGE_CURVE('',#4850,#4851,#3240,.T.);
#6337=EDGE_CURVE('',#4851,#4849,#2569,.T.);
#6338=EDGE_CURVE('',#4848,#4850,#2570,.T.);
#6339=EDGE_CURVE('',#4852,#4853,#3241,.T.);
#6340=EDGE_CURVE('',#4853,#4851,#2571,.T.);
#6341=EDGE_CURVE('',#4850,#4852,#2572,.T.);
#6342=EDGE_CURVE('',#4854,#4855,#3242,.T.);
#6343=EDGE_CURVE('',#4855,#4853,#2573,.T.);
#6344=EDGE_CURVE('',#4852,#4854,#2574,.T.);
#6345=EDGE_CURVE('',#4856,#4857,#3243,.T.);
#6346=EDGE_CURVE('',#4857,#4855,#2575,.T.);
#6347=EDGE_CURVE('',#4854,#4856,#2576,.T.);
#6348=EDGE_CURVE('',#4858,#4859,#3244,.T.);
#6349=EDGE_CURVE('',#4859,#4857,#2577,.T.);
#6350=EDGE_CURVE('',#4856,#4858,#2578,.T.);
#6351=EDGE_CURVE('',#4860,#4861,#3245,.T.);
#6352=EDGE_CURVE('',#4860,#4862,#2579,.T.);
#6353=EDGE_CURVE('',#4863,#4862,#1950,.T.);
#6354=EDGE_CURVE('',#4863,#4861,#2580,.T.);
#6355=EDGE_CURVE('',#4864,#4865,#3246,.T.);
#6356=EDGE_CURVE('',#4865,#4866,#2581,.T.);
#6357=EDGE_CURVE('',#4867,#4866,#1951,.T.);
#6358=EDGE_CURVE('',#4864,#4867,#2582,.T.);
#6359=EDGE_CURVE('',#4868,#4869,#3247,.T.);
#6360=EDGE_CURVE('',#4869,#4865,#2583,.T.);
#6361=EDGE_CURVE('',#4868,#4864,#2584,.T.);
#6362=EDGE_CURVE('',#4870,#4871,#3248,.T.);
#6363=EDGE_CURVE('',#4871,#4869,#2585,.T.);
#6364=EDGE_CURVE('',#4870,#4868,#2586,.T.);
#6365=EDGE_CURVE('',#4872,#4873,#3249,.T.);
#6366=EDGE_CURVE('',#4873,#4871,#2587,.T.);
#6367=EDGE_CURVE('',#4872,#4870,#2588,.T.);
#6368=EDGE_CURVE('',#4874,#4875,#3250,.T.);
#6369=EDGE_CURVE('',#4875,#4873,#2589,.T.);
#6370=EDGE_CURVE('',#4874,#4872,#2590,.T.);
#6371=EDGE_CURVE('',#4876,#4877,#3251,.T.);
#6372=EDGE_CURVE('',#4877,#4875,#2591,.T.);
#6373=EDGE_CURVE('',#4876,#4874,#2592,.T.);
#6374=EDGE_CURVE('',#4878,#4879,#3252,.T.);
#6375=EDGE_CURVE('',#4879,#4877,#2593,.T.);
#6376=EDGE_CURVE('',#4878,#4876,#2594,.T.);
#6377=EDGE_CURVE('',#4880,#4881,#3253,.T.);
#6378=EDGE_CURVE('',#4881,#4879,#2595,.T.);
#6379=EDGE_CURVE('',#4880,#4878,#2596,.T.);
#6380=EDGE_CURVE('',#4882,#4883,#3254,.T.);
#6381=EDGE_CURVE('',#4883,#4881,#2597,.T.);
#6382=EDGE_CURVE('',#4882,#4880,#2598,.T.);
#6383=EDGE_CURVE('',#4884,#4885,#3255,.T.);
#6384=EDGE_CURVE('',#4886,#4884,#2599,.T.);
#6385=EDGE_CURVE('',#4887,#4886,#1952,.T.);
#6386=EDGE_CURVE('',#4887,#4885,#2600,.T.);
#6387=EDGE_CURVE('',#4840,#4867,#2601,.T.);
#6388=EDGE_CURVE('',#4866,#4843,#2602,.T.);
#6389=EDGE_CURVE('',#4885,#4883,#2603,.T.);
#6390=EDGE_CURVE('',#4884,#4882,#2604,.T.);
#6391=EDGE_CURVE('',#4862,#4887,#2605,.T.);
#6392=EDGE_CURVE('',#4858,#4860,#2606,.T.);
#6393=EDGE_CURVE('',#4861,#4859,#2607,.T.);
#6394=EDGE_CURVE('',#4886,#4863,#2608,.T.);
#6395=EDGE_CURVE('',#4888,#4888,#1953,.T.);
#6396=EDGE_CURVE('',#4888,#4889,#3256,.T.);
#6397=EDGE_CURVE('',#4889,#4889,#1954,.T.);
#6398=EDGE_CURVE('',#4890,#4891,#3257,.T.);
#6399=EDGE_CURVE('',#4891,#4892,#3258,.T.);
#6400=EDGE_CURVE('',#4893,#4892,#3259,.T.);
#6401=EDGE_CURVE('',#4890,#4893,#3260,.T.);
#6402=EDGE_CURVE('',#4894,#4895,#3261,.T.);
#6403=EDGE_CURVE('',#4891,#4894,#3262,.T.);
#6404=EDGE_CURVE('',#4895,#4890,#3263,.T.);
#6405=EDGE_CURVE('',#4892,#4896,#3264,.T.);
#6406=EDGE_CURVE('',#4897,#4894,#3265,.T.);
#6407=EDGE_CURVE('',#4897,#4898,#3266,.T.);
#6408=EDGE_CURVE('',#4898,#4896,#3267,.T.);
#6409=EDGE_CURVE('',#4899,#4895,#3268,.T.);
#6410=EDGE_CURVE('',#4899,#4897,#3269,.T.);
#6411=EDGE_CURVE('',#4900,#4893,#3270,.T.);
#6412=EDGE_CURVE('',#4901,#4900,#3271,.T.);
#6413=EDGE_CURVE('',#4901,#4899,#3272,.T.);
#6414=EDGE_CURVE('',#4898,#4901,#3273,.T.);
#6415=EDGE_CURVE('',#4896,#4900,#3274,.T.);
#9101=ORIENTED_EDGE('',*,*,#6320,.T.);
#9102=ORIENTED_EDGE('',*,*,#6321,.T.);
#9103=ORIENTED_EDGE('',*,*,#6322,.T.);
#9104=ORIENTED_EDGE('',*,*,#6323,.T.);
#9105=ORIENTED_EDGE('',*,*,#6324,.T.);
#9106=ORIENTED_EDGE('',*,*,#6323,.F.);
#9107=ORIENTED_EDGE('',*,*,#6325,.T.);
#9108=ORIENTED_EDGE('',*,*,#6326,.T.);
#9109=ORIENTED_EDGE('',*,*,#6327,.T.);
#9110=ORIENTED_EDGE('',*,*,#6328,.T.);
#9111=ORIENTED_EDGE('',*,*,#6320,.F.);
#9112=ORIENTED_EDGE('',*,*,#6329,.T.);
#9113=ORIENTED_EDGE('',*,*,#6330,.T.);
#9114=ORIENTED_EDGE('',*,*,#6331,.T.);
#9115=ORIENTED_EDGE('',*,*,#6327,.F.);
#9116=ORIENTED_EDGE('',*,*,#6332,.T.);
#9117=ORIENTED_EDGE('',*,*,#6333,.T.);
#9118=ORIENTED_EDGE('',*,*,#6334,.T.);
#9119=ORIENTED_EDGE('',*,*,#6330,.F.);
#9120=ORIENTED_EDGE('',*,*,#6335,.T.);
#9121=ORIENTED_EDGE('',*,*,#6336,.T.);
#9122=ORIENTED_EDGE('',*,*,#6337,.T.);
#9123=ORIENTED_EDGE('',*,*,#6333,.F.);
#9124=ORIENTED_EDGE('',*,*,#6338,.T.);
#9125=ORIENTED_EDGE('',*,*,#6339,.T.);
#9126=ORIENTED_EDGE('',*,*,#6340,.T.);
#9127=ORIENTED_EDGE('',*,*,#6336,.F.);
#9128=ORIENTED_EDGE('',*,*,#6341,.T.);
#9129=ORIENTED_EDGE('',*,*,#6342,.T.);
#9130=ORIENTED_EDGE('',*,*,#6343,.T.);
#9131=ORIENTED_EDGE('',*,*,#6339,.F.);
#9132=ORIENTED_EDGE('',*,*,#6344,.T.);
#9133=ORIENTED_EDGE('',*,*,#6345,.T.);
#9134=ORIENTED_EDGE('',*,*,#6346,.T.);
#9135=ORIENTED_EDGE('',*,*,#6342,.F.);
#9136=ORIENTED_EDGE('',*,*,#6347,.T.);
#9137=ORIENTED_EDGE('',*,*,#6348,.T.);
#9138=ORIENTED_EDGE('',*,*,#6349,.T.);
#9139=ORIENTED_EDGE('',*,*,#6345,.F.);
#9140=ORIENTED_EDGE('',*,*,#6350,.T.);
#9141=ORIENTED_EDGE('',*,*,#6351,.F.);
#9142=ORIENTED_EDGE('',*,*,#6352,.T.);
#9143=ORIENTED_EDGE('',*,*,#6353,.F.);
#9144=ORIENTED_EDGE('',*,*,#6354,.T.);
#9145=ORIENTED_EDGE('',*,*,#6355,.T.);
#9146=ORIENTED_EDGE('',*,*,#6356,.T.);
#9147=ORIENTED_EDGE('',*,*,#6357,.F.);
#9148=ORIENTED_EDGE('',*,*,#6358,.F.);
#9149=ORIENTED_EDGE('',*,*,#6359,.T.);
#9150=ORIENTED_EDGE('',*,*,#6360,.T.);
#9151=ORIENTED_EDGE('',*,*,#6355,.F.);
#9152=ORIENTED_EDGE('',*,*,#6361,.F.);
#9153=ORIENTED_EDGE('',*,*,#6362,.T.);
#9154=ORIENTED_EDGE('',*,*,#6363,.T.);
#9155=ORIENTED_EDGE('',*,*,#6359,.F.);
#9156=ORIENTED_EDGE('',*,*,#6364,.F.);
#9157=ORIENTED_EDGE('',*,*,#6365,.T.);
#9158=ORIENTED_EDGE('',*,*,#6366,.T.);
#9159=ORIENTED_EDGE('',*,*,#6362,.F.);
#9160=ORIENTED_EDGE('',*,*,#6367,.F.);
#9161=ORIENTED_EDGE('',*,*,#6368,.T.);
#9162=ORIENTED_EDGE('',*,*,#6369,.T.);
#9163=ORIENTED_EDGE('',*,*,#6365,.F.);
#9164=ORIENTED_EDGE('',*,*,#6370,.F.);
#9165=ORIENTED_EDGE('',*,*,#6371,.T.);
#9166=ORIENTED_EDGE('',*,*,#6372,.T.);
#9167=ORIENTED_EDGE('',*,*,#6368,.F.);
#9168=ORIENTED_EDGE('',*,*,#6373,.F.);
#9169=ORIENTED_EDGE('',*,*,#6374,.T.);
#9170=ORIENTED_EDGE('',*,*,#6375,.T.);
#9171=ORIENTED_EDGE('',*,*,#6371,.F.);
#9172=ORIENTED_EDGE('',*,*,#6376,.F.);
#9173=ORIENTED_EDGE('',*,*,#6377,.T.);
#9174=ORIENTED_EDGE('',*,*,#6378,.T.);
#9175=ORIENTED_EDGE('',*,*,#6374,.F.);
#9176=ORIENTED_EDGE('',*,*,#6379,.F.);
#9177=ORIENTED_EDGE('',*,*,#6380,.T.);
#9178=ORIENTED_EDGE('',*,*,#6381,.T.);
#9179=ORIENTED_EDGE('',*,*,#6377,.F.);
#9180=ORIENTED_EDGE('',*,*,#6382,.F.);
#9181=ORIENTED_EDGE('',*,*,#6383,.F.);
#9182=ORIENTED_EDGE('',*,*,#6384,.F.);
#9183=ORIENTED_EDGE('',*,*,#6385,.F.);
#9184=ORIENTED_EDGE('',*,*,#6386,.T.);
#9185=ORIENTED_EDGE('',*,*,#6322,.F.);
#9186=ORIENTED_EDGE('',*,*,#6387,.T.);
#9187=ORIENTED_EDGE('',*,*,#6357,.T.);
#9188=ORIENTED_EDGE('',*,*,#6388,.T.);
#9189=ORIENTED_EDGE('',*,*,#6325,.F.);
#9190=ORIENTED_EDGE('',*,*,#6383,.T.);
#9191=ORIENTED_EDGE('',*,*,#6389,.T.);
#9192=ORIENTED_EDGE('',*,*,#6380,.F.);
#9193=ORIENTED_EDGE('',*,*,#6390,.F.);
#9194=ORIENTED_EDGE('',*,*,#6388,.F.);
#9195=ORIENTED_EDGE('',*,*,#6356,.F.);
#9196=ORIENTED_EDGE('',*,*,#6360,.F.);
#9197=ORIENTED_EDGE('',*,*,#6363,.F.);
#9198=ORIENTED_EDGE('',*,*,#6366,.F.);
#9199=ORIENTED_EDGE('',*,*,#6369,.F.);
#9200=ORIENTED_EDGE('',*,*,#6372,.F.);
#9201=ORIENTED_EDGE('',*,*,#6375,.F.);
#9202=ORIENTED_EDGE('',*,*,#6378,.F.);
#9203=ORIENTED_EDGE('',*,*,#6381,.F.);
#9204=ORIENTED_EDGE('',*,*,#6389,.F.);
#9205=ORIENTED_EDGE('',*,*,#6386,.F.);
#9206=ORIENTED_EDGE('',*,*,#6391,.F.);
#9207=ORIENTED_EDGE('',*,*,#6352,.F.);
#9208=ORIENTED_EDGE('',*,*,#6392,.F.);
#9209=ORIENTED_EDGE('',*,*,#6350,.F.);
#9210=ORIENTED_EDGE('',*,*,#6347,.F.);
#9211=ORIENTED_EDGE('',*,*,#6344,.F.);
#9212=ORIENTED_EDGE('',*,*,#6341,.F.);
#9213=ORIENTED_EDGE('',*,*,#6338,.F.);
#9214=ORIENTED_EDGE('',*,*,#6335,.F.);
#9215=ORIENTED_EDGE('',*,*,#6332,.F.);
#9216=ORIENTED_EDGE('',*,*,#6329,.F.);
#9217=ORIENTED_EDGE('',*,*,#6326,.F.);
#9218=ORIENTED_EDGE('',*,*,#6387,.F.);
#9219=ORIENTED_EDGE('',*,*,#6321,.F.);
#9220=ORIENTED_EDGE('',*,*,#6328,.F.);
#9221=ORIENTED_EDGE('',*,*,#6331,.F.);
#9222=ORIENTED_EDGE('',*,*,#6334,.F.);
#9223=ORIENTED_EDGE('',*,*,#6337,.F.);
#9224=ORIENTED_EDGE('',*,*,#6340,.F.);
#9225=ORIENTED_EDGE('',*,*,#6343,.F.);
#9226=ORIENTED_EDGE('',*,*,#6346,.F.);
#9227=ORIENTED_EDGE('',*,*,#6349,.F.);
#9228=ORIENTED_EDGE('',*,*,#6393,.F.);
#9229=ORIENTED_EDGE('',*,*,#6354,.F.);
#9230=ORIENTED_EDGE('',*,*,#6394,.F.);
#9231=ORIENTED_EDGE('',*,*,#6384,.T.);
#9232=ORIENTED_EDGE('',*,*,#6390,.T.);
#9233=ORIENTED_EDGE('',*,*,#6382,.T.);
#9234=ORIENTED_EDGE('',*,*,#6379,.T.);
#9235=ORIENTED_EDGE('',*,*,#6376,.T.);
#9236=ORIENTED_EDGE('',*,*,#6373,.T.);
#9237=ORIENTED_EDGE('',*,*,#6370,.T.);
#9238=ORIENTED_EDGE('',*,*,#6367,.T.);
#9239=ORIENTED_EDGE('',*,*,#6364,.T.);
#9240=ORIENTED_EDGE('',*,*,#6361,.T.);
#9241=ORIENTED_EDGE('',*,*,#6358,.T.);
#9242=ORIENTED_EDGE('',*,*,#6351,.T.);
#9243=ORIENTED_EDGE('',*,*,#6393,.T.);
#9244=ORIENTED_EDGE('',*,*,#6348,.F.);
#9245=ORIENTED_EDGE('',*,*,#6392,.T.);
#9246=ORIENTED_EDGE('',*,*,#6324,.F.);
#9247=ORIENTED_EDGE('',*,*,#6395,.F.);
#9248=ORIENTED_EDGE('',*,*,#6396,.T.);
#9249=ORIENTED_EDGE('',*,*,#6397,.F.);
#9250=ORIENTED_EDGE('',*,*,#6396,.F.);
#9251=ORIENTED_EDGE('',*,*,#6398,.T.);
#9252=ORIENTED_EDGE('',*,*,#6399,.T.);
#9253=ORIENTED_EDGE('',*,*,#6400,.F.);
#9254=ORIENTED_EDGE('',*,*,#6401,.F.);
#9255=ORIENTED_EDGE('',*,*,#6402,.F.);
#9256=ORIENTED_EDGE('',*,*,#6403,.F.);
#9257=ORIENTED_EDGE('',*,*,#6398,.F.);
#9258=ORIENTED_EDGE('',*,*,#6404,.F.);
#9259=ORIENTED_EDGE('',*,*,#6397,.T.);
#9260=ORIENTED_EDGE('',*,*,#6405,.F.);
#9261=ORIENTED_EDGE('',*,*,#6399,.F.);
#9262=ORIENTED_EDGE('',*,*,#6403,.T.);
#9263=ORIENTED_EDGE('',*,*,#6406,.F.);
#9264=ORIENTED_EDGE('',*,*,#6407,.T.);
#9265=ORIENTED_EDGE('',*,*,#6408,.T.);
#9266=ORIENTED_EDGE('',*,*,#6402,.T.);
#9267=ORIENTED_EDGE('',*,*,#6409,.F.);
#9268=ORIENTED_EDGE('',*,*,#6410,.T.);
#9269=ORIENTED_EDGE('',*,*,#6406,.T.);
#9270=ORIENTED_EDGE('',*,*,#6411,.F.);
#9271=ORIENTED_EDGE('',*,*,#6412,.F.);
#9272=ORIENTED_EDGE('',*,*,#6413,.T.);
#9273=ORIENTED_EDGE('',*,*,#6409,.T.);
#9274=ORIENTED_EDGE('',*,*,#6404,.T.);
#9275=ORIENTED_EDGE('',*,*,#6401,.T.);
#9276=ORIENTED_EDGE('',*,*,#6414,.T.);
#9277=ORIENTED_EDGE('',*,*,#6412,.T.);
#9278=ORIENTED_EDGE('',*,*,#6415,.F.);
#9279=ORIENTED_EDGE('',*,*,#6408,.F.);
#9280=ORIENTED_EDGE('',*,*,#6405,.T.);
#9281=ORIENTED_EDGE('',*,*,#6415,.T.);
#9282=ORIENTED_EDGE('',*,*,#6411,.T.);
#9283=ORIENTED_EDGE('',*,*,#6400,.T.);
#9284=ORIENTED_EDGE('',*,*,#6394,.T.);
#9285=ORIENTED_EDGE('',*,*,#6353,.T.);
#9286=ORIENTED_EDGE('',*,*,#6391,.T.);
#9287=ORIENTED_EDGE('',*,*,#6385,.T.);
#9288=ORIENTED_EDGE('',*,*,#6395,.T.);
#9289=ORIENTED_EDGE('',*,*,#6414,.F.);
#9290=ORIENTED_EDGE('',*,*,#6407,.F.);
#9291=ORIENTED_EDGE('',*,*,#6410,.F.);
#9292=ORIENTED_EDGE('',*,*,#6413,.F.);
#10479=CYLINDRICAL_SURFACE('',#11984,0.12645);
#10480=CYLINDRICAL_SURFACE('',#11988,0.12645);
#10481=CYLINDRICAL_SURFACE('',#11989,0.12645);
#10482=CYLINDRICAL_SURFACE('',#11990,0.12645);
#10483=CYLINDRICAL_SURFACE('',#11991,0.12645);
#10484=CYLINDRICAL_SURFACE('',#11992,0.12645);
#10485=CYLINDRICAL_SURFACE('',#11993,0.12645);
#10486=CYLINDRICAL_SURFACE('',#11994,0.12645);
#10487=CYLINDRICAL_SURFACE('',#11995,0.12645);
#10488=CYLINDRICAL_SURFACE('',#11996,0.12645);
#10489=CYLINDRICAL_SURFACE('',#11998,0.1543);
#10490=CYLINDRICAL_SURFACE('',#12000,0.1543);
#10491=CYLINDRICAL_SURFACE('',#12001,0.1543);
#10492=CYLINDRICAL_SURFACE('',#12002,0.1543);
#10493=CYLINDRICAL_SURFACE('',#12003,0.1543);
#10494=CYLINDRICAL_SURFACE('',#12004,0.1543);
#10495=CYLINDRICAL_SURFACE('',#12005,0.1543);
#10496=CYLINDRICAL_SURFACE('',#12006,0.1543);
#10497=CYLINDRICAL_SURFACE('',#12007,0.1543);
#10498=CYLINDRICAL_SURFACE('',#12008,0.1543);
#10499=CYLINDRICAL_SURFACE('',#12011,0.1543);
#10500=CYLINDRICAL_SURFACE('',#12012,0.12645);
#10501=CYLINDRICAL_SURFACE('',#12014,0.2);
#11024=ADVANCED_FACE('',(#899),#10479,.F.);
#11025=ADVANCED_FACE('',(#900),#10480,.F.);
#11026=ADVANCED_FACE('',(#901),#10481,.F.);
#11027=ADVANCED_FACE('',(#902),#10482,.F.);
#11028=ADVANCED_FACE('',(#903),#10483,.F.);
#11029=ADVANCED_FACE('',(#904),#10484,.F.);
#11030=ADVANCED_FACE('',(#905),#10485,.F.);
#11031=ADVANCED_FACE('',(#906),#10486,.F.);
#11032=ADVANCED_FACE('',(#907),#10487,.F.);
#11033=ADVANCED_FACE('',(#908),#10488,.F.);
#11034=ADVANCED_FACE('',(#909),#10489,.F.);
#11035=ADVANCED_FACE('',(#910),#10490,.F.);
#11036=ADVANCED_FACE('',(#911),#10491,.F.);
#11037=ADVANCED_FACE('',(#912),#10492,.F.);
#11038=ADVANCED_FACE('',(#913),#10493,.F.);
#11039=ADVANCED_FACE('',(#914),#10494,.F.);
#11040=ADVANCED_FACE('',(#915),#10495,.F.);
#11041=ADVANCED_FACE('',(#916),#10496,.F.);
#11042=ADVANCED_FACE('',(#917),#10497,.F.);
#11043=ADVANCED_FACE('',(#918),#10498,.F.);
#11044=ADVANCED_FACE('',(#919),#423,.T.);
#11045=ADVANCED_FACE('',(#920),#10499,.F.);
#11046=ADVANCED_FACE('',(#921),#247,.F.);
#11047=ADVANCED_FACE('',(#922),#248,.F.);
#11048=ADVANCED_FACE('',(#923),#10500,.F.);
#11049=ADVANCED_FACE('',(#924),#424,.F.);
#11050=ADVANCED_FACE('',(#925),#10501,.F.);
#11051=ADVANCED_FACE('',(#926),#425,.T.);
#11052=ADVANCED_FACE('',(#927,#317),#426,.F.);
#11053=ADVANCED_FACE('',(#928),#427,.T.);
#11054=ADVANCED_FACE('',(#929),#428,.T.);
#11055=ADVANCED_FACE('',(#930),#429,.T.);
#11056=ADVANCED_FACE('',(#931),#430,.T.);
#11057=ADVANCED_FACE('',(#932,#318,#319),#431,.T.);
#11058=ADVANCED_FACE('',(#933),#432,.F.);
#11239=CLOSED_SHELL('',(#11024,#11025,#11026,#11027,#11028,#11029,#11030,
#11031,#11032,#11033,#11034,#11035,#11036,#11037,#11038,#11039,#11040,#11041,
#11042,#11043,#11044,#11045,#11046,#11047,#11048,#11049,#11050,#11051,#11052,
#11053,#11054,#11055,#11056,#11057,#11058));
#11983=AXIS2_PLACEMENT_3D('',#34291,#13766,#13767);
#11984=AXIS2_PLACEMENT_3D('',#34292,#13768,#13769);
#11985=AXIS2_PLACEMENT_3D('',#34302,#13771,#13772);
#11986=AXIS2_PLACEMENT_3D('',#34305,#13774,#13775);
#11987=AXIS2_PLACEMENT_3D('',#34307,#13776,#13777);
#11988=AXIS2_PLACEMENT_3D('',#34318,#13778,#13779);
#11989=AXIS2_PLACEMENT_3D('',#34369,#13781,#13782);
#11990=AXIS2_PLACEMENT_3D('',#34420,#13784,#13785);
#11991=AXIS2_PLACEMENT_3D('',#34468,#13787,#13788);
#11992=AXIS2_PLACEMENT_3D('',#34516,#13790,#13791);
#11993=AXIS2_PLACEMENT_3D('',#34567,#13793,#13794);
#11994=AXIS2_PLACEMENT_3D('',#34618,#13796,#13797);
#11995=AXIS2_PLACEMENT_3D('',#34666,#13799,#13800);
#11996=AXIS2_PLACEMENT_3D('',#34717,#13802,#13803);
#11997=AXIS2_PLACEMENT_3D('',#34736,#13805,#13806);
#11998=AXIS2_PLACEMENT_3D('',#34756,#13807,#13808);
#11999=AXIS2_PLACEMENT_3D('',#34770,#13810,#13811);
#12000=AXIS2_PLACEMENT_3D('',#34780,#13812,#13813);
#12001=AXIS2_PLACEMENT_3D('',#34804,#13815,#13816);
#12002=AXIS2_PLACEMENT_3D('',#34829,#13818,#13819);
#12003=AXIS2_PLACEMENT_3D('',#34853,#13821,#13822);
#12004=AXIS2_PLACEMENT_3D('',#34878,#13824,#13825);
#12005=AXIS2_PLACEMENT_3D('',#34902,#13827,#13828);
#12006=AXIS2_PLACEMENT_3D('',#34927,#13830,#13831);
#12007=AXIS2_PLACEMENT_3D('',#34952,#13833,#13834);
#12008=AXIS2_PLACEMENT_3D('',#34976,#13836,#13837);
#12009=AXIS2_PLACEMENT_3D('',#34987,#13839,#13840);
#12010=AXIS2_PLACEMENT_3D('',#34993,#13841,#13842);
#12011=AXIS2_PLACEMENT_3D('',#35101,#13843,#13844);
#12012=AXIS2_PLACEMENT_3D('',#35812,#13845,#13846);
#12013=AXIS2_PLACEMENT_3D('',#35813,#13847,#13848);
#12014=AXIS2_PLACEMENT_3D('',#35814,#13849,#13850);
#12015=AXIS2_PLACEMENT_3D('',#35816,#13851,#13852);
#12016=AXIS2_PLACEMENT_3D('',#35819,#13854,#13855);
#12017=AXIS2_PLACEMENT_3D('',#35820,#13856,#13857);
#12018=AXIS2_PLACEMENT_3D('',#35829,#13862,#13863);
#12019=AXIS2_PLACEMENT_3D('',#35835,#13867,#13868);
#12020=AXIS2_PLACEMENT_3D('',#35843,#13873,#13874);
#12021=AXIS2_PLACEMENT_3D('',#35847,#13877,#13878);
#12022=AXIS2_PLACEMENT_3D('',#35853,#13882,#13883);
#12023=AXIS2_PLACEMENT_3D('',#35856,#13886,#13887);
#12024=AXIS2_PLACEMENT_3D('',#35857,#13888,#13889);
#13766=DIRECTION('axis',(0.,0.,1.));
#13767=DIRECTION('refdir',(1.,0.,0.));
#13768=DIRECTION('center_axis',(0.,0.,-1.));
#13769=DIRECTION('ref_axis',(1.,0.,0.));
#13770=DIRECTION('',(0.,0.,-1.));
#13771=DIRECTION('center_axis',(0.,0.,1.));
#13772=DIRECTION('ref_axis',(1.,0.,0.));
#13773=DIRECTION('',(0.,0.,-1.));
#13774=DIRECTION('center_axis',(0.,0.,1.));
#13775=DIRECTION('ref_axis',(1.,0.,0.));
#13776=DIRECTION('center_axis',(0.,0.,1.));
#13777=DIRECTION('ref_axis',(1.,0.,0.));
#13778=DIRECTION('center_axis',(0.,0.,-1.));
#13779=DIRECTION('ref_axis',(1.,0.,0.));
#13780=DIRECTION('',(0.,0.,-1.));
#13781=DIRECTION('center_axis',(0.,0.,-1.));
#13782=DIRECTION('ref_axis',(1.,0.,0.));
#13783=DIRECTION('',(0.,0.,-1.));
#13784=DIRECTION('center_axis',(0.,0.,-1.));
#13785=DIRECTION('ref_axis',(1.,0.,0.));
#13786=DIRECTION('',(0.,0.,-1.));
#13787=DIRECTION('center_axis',(0.,0.,-1.));
#13788=DIRECTION('ref_axis',(1.,0.,0.));
#13789=DIRECTION('',(0.,0.,-1.));
#13790=DIRECTION('center_axis',(0.,0.,-1.));
#13791=DIRECTION('ref_axis',(1.,0.,0.));
#13792=DIRECTION('',(0.,0.,-1.));
#13793=DIRECTION('center_axis',(0.,0.,-1.));
#13794=DIRECTION('ref_axis',(1.,0.,0.));
#13795=DIRECTION('',(0.,0.,-1.));
#13796=DIRECTION('center_axis',(0.,0.,-1.));
#13797=DIRECTION('ref_axis',(1.,0.,0.));
#13798=DIRECTION('',(0.,0.,-1.));
#13799=DIRECTION('center_axis',(0.,0.,-1.));
#13800=DIRECTION('ref_axis',(1.,0.,0.));
#13801=DIRECTION('',(0.,0.,-1.));
#13802=DIRECTION('center_axis',(0.,0.,-1.));
#13803=DIRECTION('ref_axis',(0.937367309351136,-0.348342543137946,0.));
#13804=DIRECTION('',(0.,0.,-1.));
#13805=DIRECTION('center_axis',(0.,0.,-1.));
#13806=DIRECTION('ref_axis',(1.,0.,0.));
#13807=DIRECTION('center_axis',(0.,0.,-1.));
#13808=DIRECTION('ref_axis',(1.,-4.8329028703551E-14,0.));
#13809=DIRECTION('',(1.22464679914735E-16,-5.93359662859705E-30,-1.));
#13810=DIRECTION('center_axis',(0.,0.,1.));
#13811=DIRECTION('ref_axis',(1.,-4.8329028703551E-14,0.));
#13812=DIRECTION('center_axis',(0.,0.,-1.));
#13813=DIRECTION('ref_axis',(1.,-4.8329028703551E-14,0.));
#13814=DIRECTION('',(1.22464679914735E-16,-5.93359662859705E-30,-1.));
#13815=DIRECTION('center_axis',(0.,0.,-1.));
#13816=DIRECTION('ref_axis',(1.,-4.8329028703551E-14,0.));
#13817=DIRECTION('',(1.22464679914735E-16,-5.93359662859705E-30,-1.));
#13818=DIRECTION('center_axis',(0.,0.,-1.));
#13819=DIRECTION('ref_axis',(1.,-4.8329028703551E-14,0.));
#13820=DIRECTION('',(1.22464679914735E-16,-5.93359662859705E-30,-1.));
#13821=DIRECTION('center_axis',(0.,0.,-1.));
#13822=DIRECTION('ref_axis',(1.,-4.8329028703551E-14,0.));
#13823=DIRECTION('',(1.22464679914735E-16,-5.93359662859705E-30,-1.));
#13824=DIRECTION('center_axis',(0.,0.,-1.));
#13825=DIRECTION('ref_axis',(1.,-4.8329028703551E-14,0.));
#13826=DIRECTION('',(1.22464679914735E-16,-5.93359662859705E-30,-1.));
#13827=DIRECTION('center_axis',(0.,0.,-1.));
#13828=DIRECTION('ref_axis',(1.,-4.8329028703551E-14,0.));
#13829=DIRECTION('',(1.22464679914735E-16,-5.93359662859705E-30,-1.));
#13830=DIRECTION('center_axis',(0.,0.,-1.));
#13831=DIRECTION('ref_axis',(1.,-4.8329028703551E-14,0.));
#13832=DIRECTION('',(1.22464679914735E-16,-5.93359662859705E-30,-1.));
#13833=DIRECTION('center_axis',(0.,0.,-1.));
#13834=DIRECTION('ref_axis',(1.,-4.8329028703551E-14,0.));
#13835=DIRECTION('',(1.22464679914735E-16,-5.93359662859705E-30,-1.));
#13836=DIRECTION('center_axis',(0.,0.,-1.));
#13837=DIRECTION('ref_axis',(-0.609222020738255,-0.792999703308644,0.));
#13838=DIRECTION('',(1.22464679914735E-16,-5.93359662859705E-30,-1.));
#13839=DIRECTION('center_axis',(0.,0.,-1.));
#13840=DIRECTION('ref_axis',(1.,-4.8329028703551E-14,0.));
#13841=DIRECTION('center_axis',(0.,0.,1.));
#13842=DIRECTION('ref_axis',(1.,0.,0.));
#13843=DIRECTION('center_axis',(0.,0.,-1.));
#13844=DIRECTION('ref_axis',(1.,-4.8329028703551E-14,0.));
#13845=DIRECTION('center_axis',(0.,0.,-1.));
#13846=DIRECTION('ref_axis',(1.,0.,0.));
#13847=DIRECTION('center_axis',(0.,0.,-1.));
#13848=DIRECTION('ref_axis',(1.,0.,0.));
#13849=DIRECTION('center_axis',(0.,0.,-1.));
#13850=DIRECTION('ref_axis',(1.,0.,0.));
#13851=DIRECTION('center_axis',(0.,0.,-1.));
#13852=DIRECTION('ref_axis',(1.,0.,0.));
#13853=DIRECTION('',(0.,0.,-1.));
#13854=DIRECTION('center_axis',(0.,0.,1.));
#13855=DIRECTION('ref_axis',(1.,0.,0.));
#13856=DIRECTION('center_axis',(1.,0.,0.));
#13857=DIRECTION('ref_axis',(0.,1.,0.));
#13858=DIRECTION('',(0.,1.,0.));
#13859=DIRECTION('',(0.,0.,1.));
#13860=DIRECTION('',(0.,1.,0.));
#13861=DIRECTION('',(0.,0.,1.));
#13862=DIRECTION('center_axis',(0.,0.,1.));
#13863=DIRECTION('ref_axis',(1.,0.,0.));
#13864=DIRECTION('',(0.,-1.,0.));
#13865=DIRECTION('',(-1.,0.,0.));
#13866=DIRECTION('',(1.,0.,0.));
#13867=DIRECTION('center_axis',(0.,1.,0.));
#13868=DIRECTION('ref_axis',(-1.,0.,0.));
#13869=DIRECTION('',(-1.,0.,0.));
#13870=DIRECTION('',(0.,0.,1.));
#13871=DIRECTION('',(-1.,0.,0.));
#13872=DIRECTION('',(0.,0.,1.));
#13873=DIRECTION('center_axis',(1.,0.,0.));
#13874=DIRECTION('ref_axis',(0.,1.,0.));
#13875=DIRECTION('',(0.,0.,1.));
#13876=DIRECTION('',(0.,1.,0.));
#13877=DIRECTION('center_axis',(0.,-1.,0.));
#13878=DIRECTION('ref_axis',(1.,0.,0.));
#13879=DIRECTION('',(1.,0.,0.));
#13880=DIRECTION('',(0.,0.,1.));
#13881=DIRECTION('',(1.,0.,0.));
#13882=DIRECTION('center_axis',(-1.,0.,0.));
#13883=DIRECTION('ref_axis',(0.,-1.,0.));
#13884=DIRECTION('',(0.,-1.,0.));
#13885=DIRECTION('',(0.,-1.,0.));
#13886=DIRECTION('center_axis',(0.,0.,1.));
#13887=DIRECTION('ref_axis',(1.,0.,0.));
#13888=DIRECTION('center_axis',(0.,0.,1.));
#13889=DIRECTION('ref_axis',(1.,0.,0.));
#34291=CARTESIAN_POINT('',(0.,0.,0.));
#34292=CARTESIAN_POINT('Origin',(0.,0.,3.7));
#34293=CARTESIAN_POINT('',(-0.126245375007135,3.12536796039931E-5,3.51934196736194));
#34294=CARTESIAN_POINT('',(-0.126365398388193,-0.00016976464794081,3.50565803263806));
#34295=CARTESIAN_POINT('',(-0.12645,1.54856587752183E-17,3.7));
#34296=CARTESIAN_POINT('',(-0.0958116152722475,0.0825211298936389,3.5));
#34297=CARTESIAN_POINT('Ctrl Pts',(-0.126365398388193,-0.00016976464794081,
3.50565803263806));
#34298=CARTESIAN_POINT('Ctrl Pts',(-0.126096583499468,0.0297434857833807,
3.5037720217587));
#34299=CARTESIAN_POINT('Ctrl Pts',(-0.115369380269343,0.0598134784363466,
3.50188601087935));
#34300=CARTESIAN_POINT('Ctrl Pts',(-0.0958116152722475,0.0825211298936389,
3.5));
#34301=CARTESIAN_POINT('',(-0.12645,1.54856587752183E-17,3.5));
#34302=CARTESIAN_POINT('Origin',(0.,0.,3.5));
#34303=CARTESIAN_POINT('',(-0.12645,-1.54856587752183E-17,3.4));
#34304=CARTESIAN_POINT('',(-0.12645,1.54856587752183E-17,3.7));
#34305=CARTESIAN_POINT('Origin',(0.,0.,3.4));
#34306=CARTESIAN_POINT('',(0.095993992990581,0.0826600147079878,3.5));
#34307=CARTESIAN_POINT('Origin',(0.,0.,3.5));
#34308=CARTESIAN_POINT('Ctrl Pts',(0.0959941578858439,0.0826601402795114,
3.5));
#34309=CARTESIAN_POINT('Ctrl Pts',(0.0693049284490514,0.113544181600847,
3.5025799450779));
#34310=CARTESIAN_POINT('Ctrl Pts',(0.0262885066473286,0.130447374694629,
3.5051598901558));
#34311=CARTESIAN_POINT('Ctrl Pts',(-0.0142676563835003,0.125842979166089,
3.5077398352337));
#34312=CARTESIAN_POINT('Ctrl Pts',(-0.0558709915822301,0.121119696778261,
3.51038639525932));
#34313=CARTESIAN_POINT('Ctrl Pts',(-0.0948853785622285,0.0937638222778825,
3.51303295528495));
#34314=CARTESIAN_POINT('Ctrl Pts',(-0.113475688700545,0.0562620506672719,
3.51567951531057));
#34315=CARTESIAN_POINT('Ctrl Pts',(-0.122051112249405,0.0389630614088429,
3.51690033266103));
#34316=CARTESIAN_POINT('Ctrl Pts',(-0.126280629837482,0.0195051929476654,
3.51812115001148));
#34317=CARTESIAN_POINT('Ctrl Pts',(-0.126245375007135,3.12536796039931E-5,
3.51934196736194));
#34318=CARTESIAN_POINT('Origin',(0.,0.,3.7));
#34319=CARTESIAN_POINT('',(-0.126440375727766,-0.00011573372396179,3.56934196736194));
#34320=CARTESIAN_POINT('',(-0.126657922659285,8.80032312977707E-6,3.55565803263806));
#34321=CARTESIAN_POINT('',(-0.12645,1.54856587752183E-17,3.7));
#34322=CARTESIAN_POINT('Ctrl Pts',(-0.126657922659285,8.80032312977707E-6,
3.55565803263806));
#34323=CARTESIAN_POINT('Ctrl Pts',(-0.126658305335383,0.00043204034557634,
3.55563127527141));
#34324=CARTESIAN_POINT('Ctrl Pts',(-0.126656367352663,0.000855276509828617,
3.55560451790477));
#34325=CARTESIAN_POINT('Ctrl Pts',(-0.126652098121077,0.00127848889899514,
3.55557776053813));
#34326=CARTESIAN_POINT('Ctrl Pts',(-0.126229830197349,0.0431382506048763,
3.5529312005125));
#34327=CARTESIAN_POINT('Ctrl Pts',(-0.103000707566798,0.0847654181274417,
3.55028464048688));
#34328=CARTESIAN_POINT('Ctrl Pts',(-0.0675987137490504,0.107109477361251,
3.54763808046125));
#34329=CARTESIAN_POINT('Ctrl Pts',(-0.0321967199313031,0.12945353659506,
3.54499152043563));
#34330=CARTESIAN_POINT('Ctrl Pts',(0.0153781450736419,0.132514487540114,
3.54234496041));
#34331=CARTESIAN_POINT('Ctrl Pts',(0.0533465621421041,0.114879483210429,
3.53969840038438));
#34332=CARTESIAN_POINT('Ctrl Pts',(0.0913149792105665,0.097244478880744,
3.53705184035875));
#34333=CARTESIAN_POINT('Ctrl Pts',(0.119676948342547,0.0589135192763201,
3.53440528033313));
#34334=CARTESIAN_POINT('Ctrl Pts',(0.125448844532432,0.0174567066922002,
3.5317587203075));
#34335=CARTESIAN_POINT('Ctrl Pts',(0.131220740722318,-0.0240001058919198,
3.52911216028188));
#34336=CARTESIAN_POINT('Ctrl Pts',(0.11440256397011,-0.0685827714557354,
3.52646560025625));
#34337=CARTESIAN_POINT('Ctrl Pts',(0.0826932442631274,-0.0959262477461666,
3.52381904023063));
#34338=CARTESIAN_POINT('Ctrl Pts',(0.0509839245561443,-0.123269724036598,
3.521172480205));
#34339=CARTESIAN_POINT('Ctrl Pts',(0.00438346189438567,-0.133374011053645,
3.51852592017938));
#34340=CARTESIAN_POINT('Ctrl Pts',(-0.0357753168513136,-0.121524408044806,
3.51587936015375));
#34341=CARTESIAN_POINT('Ctrl Pts',(-0.0759340955970119,-0.109674805035968,
3.51323280012813));
#34342=CARTESIAN_POINT('Ctrl Pts',(-0.109651190426652,-0.0758713120012468,
3.5105862401025));
#34343=CARTESIAN_POINT('Ctrl Pts',(-0.121481718337573,-0.0357885021759826,
3.50793968007688));
#34344=CARTESIAN_POINT('Ctrl Pts',(-0.124881489291372,-0.0242697961962776,
3.5071791309306));
#34345=CARTESIAN_POINT('Ctrl Pts',(-0.126473800166976,-0.012232524903913,
3.50641858178433));
#34346=CARTESIAN_POINT('Ctrl Pts',(-0.126365398388193,-0.00016976464794081,
3.50565803263806));
#34347=CARTESIAN_POINT('Ctrl Pts',(-0.126245375007135,3.12536796039931E-5,
3.51934196736194));
#34348=CARTESIAN_POINT('Ctrl Pts',(-0.12620420233203,-0.0227115638743483,
3.52076771003711));
#34349=CARTESIAN_POINT('Ctrl Pts',(-0.120346328214258,-0.0454763003201931,
3.52219345271228));
#34350=CARTESIAN_POINT('Ctrl Pts',(-0.108800985171859,-0.06484981090145,
3.52361919538745));
#34351=CARTESIAN_POINT('Ctrl Pts',(-0.0873697382082225,-0.100812232138721,
3.52626575541307));
#34352=CARTESIAN_POINT('Ctrl Pts',(-0.0463410109843132,-0.125089405892421,
3.5289123154387));
#34353=CARTESIAN_POINT('Ctrl Pts',(-0.0045038827259274,-0.126577024986295,
3.53155887546432));
#34354=CARTESIAN_POINT('Ctrl Pts',(0.0373332455324584,-0.128064644080169,
3.53420543548995));
#34355=CARTESIAN_POINT('Ctrl Pts',(0.0799787748253208,-0.106762708514216,
3.53685199551558));
#34356=CARTESIAN_POINT('Ctrl Pts',(0.103913443798274,-0.0724181339568129,
3.5394985555412));
#34357=CARTESIAN_POINT('Ctrl Pts',(0.127848112771228,-0.0380735593994097,
3.54214511556683));
#34358=CARTESIAN_POINT('Ctrl Pts',(0.133071921424273,0.00931365414944368,
3.54479167559245));
#34359=CARTESIAN_POINT('Ctrl Pts',(0.117191739814205,0.0480476856196858,
3.54743823561807));
#34360=CARTESIAN_POINT('Ctrl Pts',(0.101311558204136,0.086781717089928,
3.5500847956437));
#34361=CARTESIAN_POINT('Ctrl Pts',(0.0643273863309551,0.116862566481559,
3.55273135566933));
#34362=CARTESIAN_POINT('Ctrl Pts',(0.0231710436075753,0.124520839933968,
3.55537791569495));
#34363=CARTESIAN_POINT('Ctrl Pts',(-0.0179852991158045,0.132179113386376,
3.55802447572058));
#34364=CARTESIAN_POINT('Ctrl Pts',(-0.0633138126893829,0.117414810899563,
3.5606710357462));
#34365=CARTESIAN_POINT('Ctrl Pts',(-0.0920640726196609,0.0869862082349088,
3.56331759577183));
#34366=CARTESIAN_POINT('Ctrl Pts',(-0.113878836874053,0.0638979719779231,
3.5653257196352));
#34367=CARTESIAN_POINT('Ctrl Pts',(-0.126149033113671,0.0317913564834069,
3.56733384349857));
#34368=CARTESIAN_POINT('Ctrl Pts',(-0.126440375727766,-0.00011573372396179,
3.56934196736194));
#34369=CARTESIAN_POINT('Origin',(0.,0.,3.7));
#34370=CARTESIAN_POINT('',(-0.126640903602401,4.27927297787234E-5,3.61934196736194));
#34371=CARTESIAN_POINT('',(-0.126360536148104,0.000106176725758032,3.60565803263806));
#34372=CARTESIAN_POINT('',(-0.12645,1.54856587752183E-17,3.7));
#34373=CARTESIAN_POINT('Ctrl Pts',(-0.126360536148104,0.000106176725758032,
3.60565803263806));
#34374=CARTESIAN_POINT('Ctrl Pts',(-0.126463554653562,0.0130615819764901,
3.6048439687585));
#34375=CARTESIAN_POINT('Ctrl Pts',(-0.124630630169346,0.0259885352839278,
3.60402990487894));
#34376=CARTESIAN_POINT('Ctrl Pts',(-0.120740583509641,0.0382635675762761,
3.60321584099939));
#34377=CARTESIAN_POINT('Ctrl Pts',(-0.108093858546251,0.0781702758752103,
3.60056928097376));
#34378=CARTESIAN_POINT('Ctrl Pts',(-0.0737047770896513,0.111186630609157,
3.59792272094814));
#34379=CARTESIAN_POINT('Ctrl Pts',(-0.0333162689132352,0.122198227017938,
3.59527616092251));
#34380=CARTESIAN_POINT('Ctrl Pts',(0.00707223926318085,0.133209823426719,
3.59262960089688));
#34381=CARTESIAN_POINT('Ctrl Pts',(0.0534601741594139,0.122216661510335,
3.58998304087126));
#34382=CARTESIAN_POINT('Ctrl Pts',(0.0846116648984234,0.0942510766887394,
3.58733648084563));
#34383=CARTESIAN_POINT('Ctrl Pts',(0.115763155637433,0.0662854918671437,
3.58468992082001));
#34384=CARTESIAN_POINT('Ctrl Pts',(0.131678202219219,0.0213474841403372,
3.58204336079438));
#34385=CARTESIAN_POINT('Ctrl Pts',(0.125071080316048,-0.0199904290876357,
3.57939680076876));
#34386=CARTESIAN_POINT('Ctrl Pts',(0.118463958412876,-0.0613283423156084,
3.57675024074313));
#34387=CARTESIAN_POINT('Ctrl Pts',(0.0893346680247476,-0.0990661610447472,
3.57410368071751));
#34388=CARTESIAN_POINT('Ctrl Pts',(0.0510182611448099,-0.115928737877881,
3.57145712069188));
#34389=CARTESIAN_POINT('Ctrl Pts',(0.0127018542648722,-0.132791314711016,
3.56881056066626));
#34390=CARTESIAN_POINT('Ctrl Pts',(-0.0348016691068745,-0.128778649648146,
3.56616400064063));
#34391=CARTESIAN_POINT('Ctrl Pts',(-0.069745724184294,-0.105726139172113,
3.56351744061501));
#34392=CARTESIAN_POINT('Ctrl Pts',(-0.104336486351438,-0.0829066951932904,
3.56089763795602));
#34393=CARTESIAN_POINT('Ctrl Pts',(-0.126620455001409,-0.0414304545565597,
3.55827783529704));
#34394=CARTESIAN_POINT('Ctrl Pts',(-0.126657922659285,8.80032312977707E-6,
3.55565803263806));
#34395=CARTESIAN_POINT('Ctrl Pts',(-0.126440375727766,-0.00011573372396179,
3.56934196736194));
#34396=CARTESIAN_POINT('Ctrl Pts',(-0.126533001319164,-0.0102598491305144,
3.5699804035242));
#34397=CARTESIAN_POINT('Ctrl Pts',(-0.125414835808849,-0.020383797044434,
3.57061883968645));
#34398=CARTESIAN_POINT('Ctrl Pts',(-0.123007652953296,-0.0301913583035261,
3.5712572758487));
#34399=CARTESIAN_POINT('Ctrl Pts',(-0.113028967069674,-0.0708474193348126,
3.57390383587433));
#34400=CARTESIAN_POINT('Ctrl Pts',(-0.0808995890154535,-0.10606663855489,
3.57655039589995));
#34401=CARTESIAN_POINT('Ctrl Pts',(-0.0413281018804841,-0.119726229337694,
3.57919695592558));
#34402=CARTESIAN_POINT('Ctrl Pts',(-0.00175661474551533,-0.133385820120498,
3.5818435159512));
#34403=CARTESIAN_POINT('Ctrl Pts',(0.0452569814702019,-0.125485782466029,
3.58449007597683));
#34404=CARTESIAN_POINT('Ctrl Pts',(0.0781904578005954,-0.0996425759257176,
3.58713663600245));
#34405=CARTESIAN_POINT('Ctrl Pts',(0.111123934130988,-0.0737993693854069,
3.58978319602808));
#34406=CARTESIAN_POINT('Ctrl Pts',(0.129977290576058,-0.0300129939592548,
3.5924297560537));
#34407=CARTESIAN_POINT('Ctrl Pts',(0.126119643637387,0.0116716003968688,
3.59507631607933));
#34408=CARTESIAN_POINT('Ctrl Pts',(0.122261996698715,0.0533561947529935,
3.59772287610496));
#34409=CARTESIAN_POINT('Ctrl Pts',(0.0956933463762995,0.0929390080390894,
3.60036943613058));
#34410=CARTESIAN_POINT('Ctrl Pts',(0.0585765347711879,0.112299501333378,
3.60301599615621));
#34411=CARTESIAN_POINT('Ctrl Pts',(0.0214597231660768,0.131659994627667,
3.60566255618183));
#34412=CARTESIAN_POINT('Ctrl Pts',(-0.0262052497217305,0.130798167930148,
3.60830911620746));
#34413=CARTESIAN_POINT('Ctrl Pts',(-0.0625979093128853,0.11010854389779,
3.61095567623308));
#34414=CARTESIAN_POINT('Ctrl Pts',(-0.0989905689040401,0.089418919865431,
3.61360223625871));
#34415=CARTESIAN_POINT('Ctrl Pts',(-0.124110915198542,0.048901498498232,
3.61624879628433));
#34416=CARTESIAN_POINT('Ctrl Pts',(-0.12645913501461,0.00710470077718534,
3.61889535630996));
#34417=CARTESIAN_POINT('Ctrl Pts',(-0.126591223576389,0.00475360959731907,
3.61904422666062));
#34418=CARTESIAN_POINT('Ctrl Pts',(-0.126651258400685,0.00239847031733228,
3.61919309701128));
#34419=CARTESIAN_POINT('Ctrl Pts',(-0.126640903602401,4.27927297787234E-5,
3.61934196736194));
#34420=CARTESIAN_POINT('Origin',(0.,0.,3.7));
#34421=CARTESIAN_POINT('',(-0.126313625852874,8.92012377725487E-5,3.66934196736194));
#34422=CARTESIAN_POINT('',(-0.126280524269743,-6.82698929511343E-5,3.65565803263806));
#34423=CARTESIAN_POINT('',(-0.12645,1.54856587752183E-17,3.7));
#34424=CARTESIAN_POINT('Ctrl Pts',(-0.126280524269743,-6.82698929511343E-5,
3.65565803263806));
#34425=CARTESIAN_POINT('Ctrl Pts',(-0.126155459137289,0.0254573418705088,
3.65405666224558));
#34426=CARTESIAN_POINT('Ctrl Pts',(-0.1186500792639,0.0510505822956786,
3.65245529185311));
#34427=CARTESIAN_POINT('Ctrl Pts',(-0.104270310346229,0.0719033403784211,
3.65085392146064));
#34428=CARTESIAN_POINT('Ctrl Pts',(-0.0805050891493468,0.106366370433962,
3.64820736143502));
#34429=CARTESIAN_POINT('Ctrl Pts',(-0.0379633950684185,0.127881407935326,
3.64556080140939));
#34430=CARTESIAN_POINT('Ctrl Pts',(0.00387966794034225,0.126599115215449,
3.64291424138376));
#34431=CARTESIAN_POINT('Ctrl Pts',(0.0457227309491033,0.125316822495572,
3.64026768135814));
#34432=CARTESIAN_POINT('Ctrl Pts',(0.0868671628856968,0.101237199554454,
3.63762112133251));
#34433=CARTESIAN_POINT('Ctrl Pts',(0.108477510477425,0.0653836202783246,
3.63497456130689));
#34434=CARTESIAN_POINT('Ctrl Pts',(0.130087858069152,0.0295300410021955,
3.63232800128126));
#34435=CARTESIAN_POINT('Ctrl Pts',(0.132164121316015,-0.018097494608945,
3.62968144125564));
#34436=CARTESIAN_POINT('Ctrl Pts',(0.113755810560665,-0.0556956347668708,
3.62703488123001));
#34437=CARTESIAN_POINT('Ctrl Pts',(0.0953474998053144,-0.0932937749247968,
3.62438832120439));
#34438=CARTESIAN_POINT('Ctrl Pts',(0.0564546150477511,-0.120862519629508,
3.62174176117876));
#34439=CARTESIAN_POINT('Ctrl Pts',(0.0148818767183724,-0.125781225334577,
3.61909520115314));
#34440=CARTESIAN_POINT('Ctrl Pts',(-0.0266908616110063,-0.130699931039647,
3.61644864112751));
#34441=CARTESIAN_POINT('Ctrl Pts',(-0.0709434535122003,-0.112968597745074,
3.61380208110189));
#34442=CARTESIAN_POINT('Ctrl Pts',(-0.0976175652277067,-0.0807044001658271,
3.61115552107626));
#34443=CARTESIAN_POINT('Ctrl Pts',(-0.116086901439685,-0.0583644505151555,
3.60932302493019));
#34444=CARTESIAN_POINT('Ctrl Pts',(-0.126128636638782,-0.0290570508647223,
3.60749052878412));
#34445=CARTESIAN_POINT('Ctrl Pts',(-0.126360536148104,0.000106176725758032,
3.60565803263806));
#34446=CARTESIAN_POINT('Ctrl Pts',(-0.126640903602401,4.27927297787234E-5,
3.61934196736194));
#34447=CARTESIAN_POINT('Ctrl Pts',(-0.126467174766239,-0.0394798628014113,
3.62183965703691));
#34448=CARTESIAN_POINT('Ctrl Pts',(-0.106479582237496,-0.0791540456794125,
3.62433734671187));
#34449=CARTESIAN_POINT('Ctrl Pts',(-0.0745372494842149,-0.102404041708738,
3.62683503638683));
#34450=CARTESIAN_POINT('Ctrl Pts',(-0.0406910508001211,-0.12703981239872,
3.62948159641246));
#34451=CARTESIAN_POINT('Ctrl Pts',(0.00657743990569856,-0.133235179703789,
3.63212815643808));
#34452=CARTESIAN_POINT('Ctrl Pts',(0.0456292459986054,-0.118153973308938,
3.63477471646371));
#34453=CARTESIAN_POINT('Ctrl Pts',(0.0846810520915122,-0.103072766914087,
3.63742127648934));
#34454=CARTESIAN_POINT('Ctrl Pts',(0.115516173571506,-0.0667149868193161,
3.64006783651496));
#34455=CARTESIAN_POINT('Ctrl Pts',(0.124018641769873,-0.0257248122789798,
3.64271439654059));
#34456=CARTESIAN_POINT('Ctrl Pts',(0.132521109968241,0.0152653622613568,
3.64536095656621));
#34457=CARTESIAN_POINT('Ctrl Pts',(0.11869092488498,0.0608879312472584,
3.64800751659183));
#34458=CARTESIAN_POINT('Ctrl Pts',(0.0888593883296617,0.0902574016134864,
3.65065407661746));
#34459=CARTESIAN_POINT('Ctrl Pts',(0.0590278517743432,0.119626871979714,
3.65330063664309));
#34460=CARTESIAN_POINT('Ctrl Pts',(0.0131949637469664,0.132743243726269,
3.65594719666871));
#34461=CARTESIAN_POINT('Ctrl Pts',(-0.027657500752443,0.123601990750641,
3.65859375669434));
#34462=CARTESIAN_POINT('Ctrl Pts',(-0.0685099652518527,0.114460737775013,
3.66124031671997));
#34463=CARTESIAN_POINT('Ctrl Pts',(-0.104382006223295,0.0830618600772021,
3.66388687674559));
#34464=CARTESIAN_POINT('Ctrl Pts',(-0.118851810998494,0.043779407059542,
3.66653343677121));
#34465=CARTESIAN_POINT('Ctrl Pts',(-0.123970265263591,0.0298838886116103,
3.66746961363479));
#34466=CARTESIAN_POINT('Ctrl Pts',(-0.126410714036168,0.0150019191305398,
3.66840579049837));
#34467=CARTESIAN_POINT('Ctrl Pts',(-0.126313625852874,8.92012377725487E-5,
3.66934196736194));
#34468=CARTESIAN_POINT('Origin',(0.,0.,3.7));
#34469=CARTESIAN_POINT('',(-0.126318202311182,-9.13759226411071E-5,3.71934196736194));
#34470=CARTESIAN_POINT('',(-0.126609590382811,-7.02044759900073E-5,3.70565803263806));
#34471=CARTESIAN_POINT('',(-0.12645,1.54856587752183E-17,3.7));
#34472=CARTESIAN_POINT('Ctrl Pts',(-0.126609590382811,-7.02044759900073E-5,
3.70565803263806));
#34473=CARTESIAN_POINT('Ctrl Pts',(-0.126357411318116,0.0377522139233435,
3.70326935573267));
#34474=CARTESIAN_POINT('Ctrl Pts',(-0.108290467899376,0.0757836426892297,
3.70088067882728));
#34475=CARTESIAN_POINT('Ctrl Pts',(-0.0786816086433086,0.099255188273642,
3.6984920019219));
#34476=CARTESIAN_POINT('Ctrl Pts',(-0.0458761575859702,0.125260737263231,
3.69584544189627));
#34477=CARTESIAN_POINT('Ctrl Pts',(0.00109788169852634,0.133392911300054,
3.69319888187064));
#34478=CARTESIAN_POINT('Ctrl Pts',(0.0407363279886946,0.119928893584969,
3.69055232184502));
#34479=CARTESIAN_POINT('Ctrl Pts',(0.0803747742788628,0.106464875869883,
3.68790576181939));
#34480=CARTESIAN_POINT('Ctrl Pts',(0.112677627574703,0.071404666402888,
3.68525920179377));
#34481=CARTESIAN_POINT('Ctrl Pts',(0.122857008829439,0.0307984304737455,
3.68261264176814));
#34482=CARTESIAN_POINT('Ctrl Pts',(0.133036390084175,-0.00980780545539708,
3.67996608174252));
#34483=CARTESIAN_POINT('Ctrl Pts',(0.121092299297808,-0.0559600678466875,
3.67731952171689));
#34484=CARTESIAN_POINT('Ctrl Pts',(0.0924926054626293,-0.08653037546552,
3.67467296169127));
#34485=CARTESIAN_POINT('Ctrl Pts',(0.0638929116274508,-0.117100683084353,
3.67202640166564));
#34486=CARTESIAN_POINT('Ctrl Pts',(0.0186376147434612,-0.132089035930727,
3.66937984164002));
#34487=CARTESIAN_POINT('Ctrl Pts',(-0.0225559247032424,-0.124633936707157,
3.66673328161439));
#34488=CARTESIAN_POINT('Ctrl Pts',(-0.063749464149946,-0.117178837483586,
3.66408672158877));
#34489=CARTESIAN_POINT('Ctrl Pts',(-0.100881246159364,-0.0872802861900701,
3.66144016156314));
#34490=CARTESIAN_POINT('Ctrl Pts',(-0.116952763007655,-0.0486254992384533,
3.65879360153752));
#34491=CARTESIAN_POINT('Ctrl Pts',(-0.123299788065177,-0.0333598025596003,
3.65774841190436));
#34492=CARTESIAN_POINT('Ctrl Pts',(-0.126362152343126,-0.016728441031668,
3.65670322227121));
#34493=CARTESIAN_POINT('Ctrl Pts',(-0.126280524269743,-6.82698929511343E-5,
3.65565803263806));
#34494=CARTESIAN_POINT('Ctrl Pts',(-0.126313625852874,8.92012377725487E-5,
3.66934196736194));
#34495=CARTESIAN_POINT('Ctrl Pts',(-0.126136246983132,-0.027156143714207,
3.67105235052399));
#34496=CARTESIAN_POINT('Ctrl Pts',(-0.117488868450918,-0.0545041232450019,
3.67276273368604));
#34497=CARTESIAN_POINT('Ctrl Pts',(-0.101228105076468,-0.0761266063810683,
3.67447311684809));
#34498=CARTESIAN_POINT('Ctrl Pts',(-0.0760670258002872,-0.10958413846651,
3.67711967687372));
#34499=CARTESIAN_POINT('Ctrl Pts',(-0.0326772986689716,-0.129333174299883,
3.67976623689934));
#34500=CARTESIAN_POINT('Ctrl Pts',(0.00907775247578101,-0.126332829739009,
3.68241279692497));
#34501=CARTESIAN_POINT('Ctrl Pts',(0.050832803620533,-0.123332485178135,
3.68505935695059));
#34502=CARTESIAN_POINT('Ctrl Pts',(0.0909531787787221,-0.0975827602230137,
3.68770591697622));
#34503=CARTESIAN_POINT('Ctrl Pts',(0.11107222624856,-0.0608715862708329,
3.69035247700184));
#34504=CARTESIAN_POINT('Ctrl Pts',(0.131191273718398,-0.0241604123186516,
3.69299903702747));
#34505=CARTESIAN_POINT('Ctrl Pts',(0.131308993499885,0.0235122106305895,
3.69564559705309));
#34506=CARTESIAN_POINT('Ctrl Pts',(0.111371494820412,0.0603222977018694,
3.69829215707872));
#34507=CARTESIAN_POINT('Ctrl Pts',(0.0914339961409399,0.097132384773149,
3.70093871710434));
#34508=CARTESIAN_POINT('Ctrl Pts',(0.0514412790005074,0.123079935966467,
3.70358527712997));
#34509=CARTESIAN_POINT('Ctrl Pts',(0.00970155469863815,0.126286457292336,
3.70623183715559));
#34510=CARTESIAN_POINT('Ctrl Pts',(-0.0320381696032317,0.129492978618205,
3.70887839718122));
#34511=CARTESIAN_POINT('Ctrl Pts',(-0.0755249010665388,0.109958470076624,
3.71152495720684));
#34512=CARTESIAN_POINT('Ctrl Pts',(-0.100850908347825,0.0766256076274997,
3.71417151723247));
#34513=CARTESIAN_POINT('Ctrl Pts',(-0.117343620441844,0.0549186998809637,
3.71589500060896));
#34514=CARTESIAN_POINT('Ctrl Pts',(-0.126134681028771,0.0273601470071565,
3.71761848398545));
#34515=CARTESIAN_POINT('Ctrl Pts',(-0.126318202311182,-9.13759226411071E-5,
3.71934196736194));
#34516=CARTESIAN_POINT('Origin',(0.,0.,3.7));
#34517=CARTESIAN_POINT('',(-0.126643738265873,-3.92119282522094E-5,3.76934196736194));
#34518=CARTESIAN_POINT('',(-0.126492921331233,0.000111898061355794,3.75565803263806));
#34519=CARTESIAN_POINT('',(-0.12645,1.54856587752183E-17,3.7));
#34520=CARTESIAN_POINT('Ctrl Pts',(-0.126492921331233,0.000111898061355794,
3.75565803263806));
#34521=CARTESIAN_POINT('Ctrl Pts',(-0.12657025228906,0.00851493641555574,
3.75512860924538));
#34522=CARTESIAN_POINT('Ctrl Pts',(-0.125804504023154,0.0169039539351017,
3.7545991858527));
#34523=CARTESIAN_POINT('Ctrl Pts',(-0.12414416907011,0.0251120135156184,
3.75406976246003));
#34524=CARTESIAN_POINT('Ctrl Pts',(-0.115844240928182,0.06614367678216,
3.7514232024344));
#34525=CARTESIAN_POINT('Ctrl Pts',(-0.0851890554053168,0.102653294996741,
3.74877664240878));
#34526=CARTESIAN_POINT('Ctrl Pts',(-0.0462122079706087,0.117927179951992,
3.74613008238315));
#34527=CARTESIAN_POINT('Ctrl Pts',(-0.00723536053590029,0.133201064907244,
3.74348352235752));
#34528=CARTESIAN_POINT('Ctrl Pts',(0.0400631488106516,0.127239216603166,
3.7408369623319));
#34529=CARTESIAN_POINT('Ctrl Pts',(0.0740306001411793,0.102770901424588,
3.73819040230627));
#34530=CARTESIAN_POINT('Ctrl Pts',(0.107998051471707,0.0783025862460102,
3.73554384228065));
#34531=CARTESIAN_POINT('Ctrl Pts',(0.12863444478621,0.0353278041929325,
3.73289728225502));
#34532=CARTESIAN_POINT('Ctrl Pts',(0.126492673803057,-0.00648007801438488,
3.7302507222294));
#34533=CARTESIAN_POINT('Ctrl Pts',(0.124350902819903,-0.0482879602217022,
3.72760416220377));
#34534=CARTESIAN_POINT('Ctrl Pts',(0.0994309675390923,-0.0889289425832592,
3.72495760217815));
#34535=CARTESIAN_POINT('Ctrl Pts',(0.063140931062625,-0.109798045345167,
3.72231104215252));
#34536=CARTESIAN_POINT('Ctrl Pts',(0.0268508945861577,-0.130667148107075,
3.7196644821269));
#34537=CARTESIAN_POINT('Ctrl Pts',(-0.020809243085966,-0.131764371269333,
3.71701792210127));
#34538=CARTESIAN_POINT('Ctrl Pts',(-0.0580212126891809,-0.112587418545307,
3.71437136207565));
#34539=CARTESIAN_POINT('Ctrl Pts',(-0.0952331822923957,-0.0934104658212808,
3.71172480205002));
#34540=CARTESIAN_POINT('Ctrl Pts',(-0.121996983826702,-0.0539593372109697,
3.7090782420244));
#34541=CARTESIAN_POINT('Ctrl Pts',(-0.126060453178764,-0.0122943109346363,
3.70643168199877));
#34542=CARTESIAN_POINT('Ctrl Pts',(-0.126456401181211,-0.00823443438662399,
3.70617379887853));
#34543=CARTESIAN_POINT('Ctrl Pts',(-0.126636815799491,-0.0041535374917583,
3.70591591575829));
#34544=CARTESIAN_POINT('Ctrl Pts',(-0.126609590382811,-7.02044759900073E-5,
3.70565803263806));
#34545=CARTESIAN_POINT('Ctrl Pts',(-0.126318202311182,-9.13759226411071E-5,
3.71934196736194));
#34546=CARTESIAN_POINT('Ctrl Pts',(-0.126416494068865,-0.0147940763636936,
3.72026504401107));
#34547=CARTESIAN_POINT('Ctrl Pts',(-0.12404567634908,-0.0294660748073717,
3.72118812066021));
#34548=CARTESIAN_POINT('Ctrl Pts',(-0.119066572492589,-0.0431919063448052,
3.72211119730934));
#34549=CARTESIAN_POINT('Ctrl Pts',(-0.104790946256804,-0.0825453415113195,
3.72475775733497));
#34550=CARTESIAN_POINT('Ctrl Pts',(-0.0690744106859675,-0.11412099548768,
3.7274043173606));
#34551=CARTESIAN_POINT('Ctrl Pts',(-0.0282675897675097,-0.123463892809314,
3.73005087738622));
#34552=CARTESIAN_POINT('Ctrl Pts',(0.0125392311509478,-0.132806790130948,
3.73269743741185));
#34553=CARTESIAN_POINT('Ctrl Pts',(0.0584363374170267,-0.119916930797855,
3.73534399743747));
#34554=CARTESIAN_POINT('Ctrl Pts',(0.0884125555029259,-0.0906951458916328,
3.7379905574631));
#34555=CARTESIAN_POINT('Ctrl Pts',(0.118388773588825,-0.0614733609854108,
3.74063711748872));
#34556=CARTESIAN_POINT('Ctrl Pts',(0.132444103494545,-0.0159196505060593,
3.74328367751435));
#34557=CARTESIAN_POINT('Ctrl Pts',(0.124144174958903,0.0251120147068241,
3.74593023753997));
#34558=CARTESIAN_POINT('Ctrl Pts',(0.115844246423262,0.0661436799197074,
3.7485767975656));
#34559=CARTESIAN_POINT('Ctrl Pts',(0.0851890594462595,0.102653299866123,
3.75122335759122));
#34560=CARTESIAN_POINT('Ctrl Pts',(0.0462122101626772,0.117927185545889,
3.75386991761685));
#34561=CARTESIAN_POINT('Ctrl Pts',(0.00723536087909469,0.133201071225655,
3.75651647764247));
#34562=CARTESIAN_POINT('Ctrl Pts',(-0.0400631507110678,0.127239222638772,
3.7591630376681));
#34563=CARTESIAN_POINT('Ctrl Pts',(-0.0740306036528435,0.102770906299531,
3.76180959769372));
#34564=CARTESIAN_POINT('Ctrl Pts',(-0.106255505634774,0.0795578294448588,
3.76432038758313));
#34565=CARTESIAN_POINT('Ctrl Pts',(-0.12648204772981,0.0396883664632768,
3.76683117747254));
#34566=CARTESIAN_POINT('Ctrl Pts',(-0.126643738265873,-3.92119282522094E-5,
3.76934196736194));
#34567=CARTESIAN_POINT('Origin',(0.,0.,3.7));
#34568=CARTESIAN_POINT('',(-0.12643411897368,0.000115681837355761,3.81934196736194));
#34569=CARTESIAN_POINT('',(-0.126243465328102,1.71616150689059E-6,3.80565803263806));
#34570=CARTESIAN_POINT('',(-0.12645,1.54856587752183E-17,3.7));
#34571=CARTESIAN_POINT('Ctrl Pts',(-0.126243465328102,1.71616150689059E-6,
3.80565803263806));
#34572=CARTESIAN_POINT('Ctrl Pts',(-0.126246007062352,0.0210055997219054,
3.80434130273247));
#34573=CARTESIAN_POINT('Ctrl Pts',(-0.121290894068088,0.0420083553470164,
3.80302457282688));
#34574=CARTESIAN_POINT('Ctrl Pts',(-0.111371489537494,0.0603222948404575,
3.80170784292128));
#34575=CARTESIAN_POINT('Ctrl Pts',(-0.0914339918037617,0.0971323801656441,
3.79906128289566));
#34576=CARTESIAN_POINT('Ctrl Pts',(-0.0514412765603963,0.123079930128149,
3.79641472287003));
#34577=CARTESIAN_POINT('Ctrl Pts',(-0.00970155423845781,0.126286451301922,
3.79376816284441));
#34578=CARTESIAN_POINT('Ctrl Pts',(0.0320381680834807,0.129492972475696,
3.79112160281878));
#34579=CARTESIAN_POINT('Ctrl Pts',(0.0755248974839926,0.109958464860738,
3.78847504279316));
#34580=CARTESIAN_POINT('Ctrl Pts',(0.10085090356394,0.0766256039927644,
3.78582848276753));
#34581=CARTESIAN_POINT('Ctrl Pts',(0.126176909643887,0.0432927431247909,
3.78318192274191));
#34582=CARTESIAN_POINT('Ctrl Pts',(0.13334219240327,-0.00383847099619805,
3.78053536271628));
#34583=CARTESIAN_POINT('Ctrl Pts',(0.119066566844655,-0.0431919042959778,
3.77788880269065));
#34584=CARTESIAN_POINT('Ctrl Pts',(0.10479094128604,-0.0825453375957573,
3.77524224266503));
#34585=CARTESIAN_POINT('Ctrl Pts',(0.0690744074094266,-0.114120990074327,
3.7725956826394));
#34586=CARTESIAN_POINT('Ctrl Pts',(0.0282675884266474,-0.123463886952785,
3.76994912261378));
#34587=CARTESIAN_POINT('Ctrl Pts',(-0.0125392305561318,-0.132806783831242,
3.76730256258815));
#34588=CARTESIAN_POINT('Ctrl Pts',(-0.0584363346450773,-0.119916925109586,
3.76465600256253));
#34589=CARTESIAN_POINT('Ctrl Pts',(-0.088412551309054,-0.0906951415895065,
3.7620094425369));
#34590=CARTESIAN_POINT('Ctrl Pts',(-0.112392263011044,-0.0673189446502994,
3.75989230590395));
#34591=CARTESIAN_POINT('Ctrl Pts',(-0.126183678849807,-0.0334914156074963,
3.75777516927101));
#34592=CARTESIAN_POINT('Ctrl Pts',(-0.126492921331233,0.000111898061355794,
3.75565803263806));
#34593=CARTESIAN_POINT('Ctrl Pts',(-0.126643738265873,-3.92119282522094E-5,
3.76934196736194));
#34594=CARTESIAN_POINT('Ctrl Pts',(-0.12665248162835,-0.00218746764357669,
3.76947773749816));
#34595=CARTESIAN_POINT('Ctrl Pts',(-0.126602553960315,-0.00433530847842783,
3.76961350763438));
#34596=CARTESIAN_POINT('Ctrl Pts',(-0.126492679803253,-0.0064800783217853,
3.7697492777706));
#34597=CARTESIAN_POINT('Ctrl Pts',(-0.124350908718499,-0.0482879625122638,
3.77239583779623));
#34598=CARTESIAN_POINT('Ctrl Pts',(-0.0994309722556023,-0.0889289468016232,
3.77504239782185));
#34599=CARTESIAN_POINT('Ctrl Pts',(-0.0631409340577098,-0.109798050553457,
3.77768895784748));
#34600=CARTESIAN_POINT('Ctrl Pts',(-0.0268508958598173,-0.130667154305292,
3.7803355178731));
#34601=CARTESIAN_POINT('Ctrl Pts',(0.0208092440730706,-0.131764377519601,
3.78298207789873));
#34602=CARTESIAN_POINT('Ctrl Pts',(0.0580212154414384,-0.112587423885904,
3.78562863792435));
#34603=CARTESIAN_POINT('Ctrl Pts',(0.0952331868098064,-0.0934104702522078,
3.78827519794998));
#34604=CARTESIAN_POINT('Ctrl Pts',(0.121996989613654,-0.0539593397705055,
3.7909217579756));
#34605=CARTESIAN_POINT('Ctrl Pts',(0.126060459158462,-0.0122943115177929,
3.79356831800123));
#34606=CARTESIAN_POINT('Ctrl Pts',(0.130123928703269,0.0293707167349194,
3.79621487802685));
#34607=CARTESIAN_POINT('Ctrl Pts',(0.111487064989038,0.073249642758642,
3.79886143805248));
#34608=CARTESIAN_POINT('Ctrl Pts',(0.0786816123755665,0.0992551929818185,
3.8015079980781));
#34609=CARTESIAN_POINT('Ctrl Pts',(0.0458761597620954,0.125260743204995,
3.80415455810373));
#34610=CARTESIAN_POINT('Ctrl Pts',(-0.00109788175061491,0.133392917627625,
3.80680111812935));
#34611=CARTESIAN_POINT('Ctrl Pts',(-0.0407363299210399,0.119928899273839,
3.80944767815498));
#34612=CARTESIAN_POINT('Ctrl Pts',(-0.0803747780914649,0.106464880920053,
3.81209423818061));
#34613=CARTESIAN_POINT('Ctrl Pts',(-0.112677632919605,0.071404669789851,
3.81474079820623));
#34614=CARTESIAN_POINT('Ctrl Pts',(-0.122857014657189,0.030798431934596,
3.81738735823185));
#34615=CARTESIAN_POINT('Ctrl Pts',(-0.125362998814015,0.0208018927186779,
3.81803889460855));
#34616=CARTESIAN_POINT('Ctrl Pts',(-0.126528173261855,0.0104692323861157,
3.81869043098525));
#34617=CARTESIAN_POINT('Ctrl Pts',(-0.12643411897368,0.000115681837355761,
3.81934196736194));
#34618=CARTESIAN_POINT('Origin',(0.,0.,3.7));
#34619=CARTESIAN_POINT('',(-0.126249985800877,-2.99474503126992E-5,3.86934196736194));
#34620=CARTESIAN_POINT('',(-0.126486618721746,-0.000112766438119152,3.85565803263806));
#34621=CARTESIAN_POINT('',(-0.12645,1.54856587752183E-17,3.7));
#34622=CARTESIAN_POINT('Ctrl Pts',(-0.126486618721746,-0.000112766438119152,
3.85565803263806));
#34623=CARTESIAN_POINT('Ctrl Pts',(-0.126178545401481,0.0332869000256312,
3.85355399621955));
#34624=CARTESIAN_POINT('Ctrl Pts',(-0.112575693492532,0.0669084342579941,
3.85144995980104));
#34625=CARTESIAN_POINT('Ctrl Pts',(-0.0888593841145145,0.0902573973319142,
3.84934592338254));
#34626=CARTESIAN_POINT('Ctrl Pts',(-0.0590278489741825,0.119626866304839,
3.84669936335691));
#34627=CARTESIAN_POINT('Ctrl Pts',(-0.0131949631210826,0.13274323742959,
3.84405280333129));
#34628=CARTESIAN_POINT('Ctrl Pts',(0.0276574994404428,0.123601984887668,
3.84140624330566));
#34629=CARTESIAN_POINT('Ctrl Pts',(0.0685099620019675,0.114460732345747,
3.83875968328004));
#34630=CARTESIAN_POINT('Ctrl Pts',(0.104382001271918,0.0830618561371527,
3.83611312325441));
#34631=CARTESIAN_POINT('Ctrl Pts',(0.118851805360766,0.0437794049828168,
3.83346656322878));
#34632=CARTESIAN_POINT('Ctrl Pts',(0.133321609449615,0.00449695382848087,
3.83082000320316));
#34633=CARTESIAN_POINT('Ctrl Pts',(0.126389178357361,-0.0426690722715969,
3.82817344317753));
#34634=CARTESIAN_POINT('Ctrl Pts',(0.101228100274691,-0.0761266027699533,
3.82552688315191));
#34635=CARTESIAN_POINT('Ctrl Pts',(0.0760670221920212,-0.10958413326831,
3.82288032312628));
#34636=CARTESIAN_POINT('Ctrl Pts',(0.0326772971189339,-0.129333168164945,
3.82023376310066));
#34637=CARTESIAN_POINT('Ctrl Pts',(-0.0090777520451555,-0.12633282374641,
3.81758720307503));
#34638=CARTESIAN_POINT('Ctrl Pts',(-0.0508328012092449,-0.123332479327876,
3.81494064304941));
#34639=CARTESIAN_POINT('Ctrl Pts',(-0.0909531744643365,-0.097582755594171,
3.81229408302378));
#34640=CARTESIAN_POINT('Ctrl Pts',(-0.111072220979832,-0.0608715833833843,
3.80964752299816));
#34641=CARTESIAN_POINT('Ctrl Pts',(-0.121181537898249,-0.0424251389139816,
3.80831769287812));
#34642=CARTESIAN_POINT('Ctrl Pts',(-0.126240898306005,-0.021211136130883,
3.80698786275809));
#34643=CARTESIAN_POINT('Ctrl Pts',(-0.126243465328102,1.71616150689059E-6,
3.80565803263806));
#34644=CARTESIAN_POINT('Ctrl Pts',(-0.12643411897368,0.000115681837355761,
3.81934196736194));
#34645=CARTESIAN_POINT('Ctrl Pts',(-0.126146121962456,-0.0315871960586303,
3.82133699101087));
#34646=CARTESIAN_POINT('Ctrl Pts',(-0.114051564760291,-0.0634859411452914,
3.8233320146598));
#34647=CARTESIAN_POINT('Ctrl Pts',(-0.0924926098500027,-0.0865303795699984,
3.82532703830873));
#34648=CARTESIAN_POINT('Ctrl Pts',(-0.0638929146582029,-0.117100688639029,
3.82797359833436));
#34649=CARTESIAN_POINT('Ctrl Pts',(-0.018637615627574,-0.132089042196783,
3.83062015835998));
#34650=CARTESIAN_POINT('Ctrl Pts',(0.0225559257731756,-0.124633942619396,
3.83326671838561));
#34651=CARTESIAN_POINT('Ctrl Pts',(0.0637494671739252,-0.117178843042008,
3.83591327841123));
#34652=CARTESIAN_POINT('Ctrl Pts',(0.100881250944795,-0.0872802903294789,
3.83855983843686));
#34653=CARTESIAN_POINT('Ctrl Pts',(0.116952768555385,-0.048625501544595,
3.84120639846248));
#34654=CARTESIAN_POINT('Ctrl Pts',(0.133024286165975,-0.00997071275971127,
3.84385295848811));
#34655=CARTESIAN_POINT('Ctrl Pts',(0.128035537616284,0.0374403120975275,
3.84649951851373));
#34656=CARTESIAN_POINT('Ctrl Pts',(0.10427031529219,0.0719033437884345,
3.84914607853936));
#34657=CARTESIAN_POINT('Ctrl Pts',(0.080505092968096,0.106366375479342,
3.85179263856498));
#34658=CARTESIAN_POINT('Ctrl Pts',(0.037963396869598,0.127881414003918,
3.85443919859061));
#34659=CARTESIAN_POINT('Ctrl Pts',(-0.003879668124188,0.126599121222081,
3.85708575861623));
#34660=CARTESIAN_POINT('Ctrl Pts',(-0.0457227331179738,0.125316828440245,
3.85973231864186));
#34661=CARTESIAN_POINT('Ctrl Pts',(-0.0868671670070475,0.101237204351996,
3.86237887866749));
#34662=CARTESIAN_POINT('Ctrl Pts',(-0.108477515623481,0.0653836233772192,
3.86502543869311));
#34663=CARTESIAN_POINT('Ctrl Pts',(-0.120226312608128,0.0458912749879413,
3.86646428158272));
#34664=CARTESIAN_POINT('Ctrl Pts',(-0.126201381437229,0.0229188749131541,
3.86790312447233));
#34665=CARTESIAN_POINT('Ctrl Pts',(-0.126249985800877,-2.99474503126992E-5,
3.86934196736194));
#34666=CARTESIAN_POINT('Origin',(0.,0.,3.7));
#34667=CARTESIAN_POINT('',(-0.126543984365092,-0.000100563349596846,3.91934196736194));
#34668=CARTESIAN_POINT('',(-0.126614009842867,6.71750503076223E-5,3.90565803263806));
#34669=CARTESIAN_POINT('',(-0.12645,1.54856587752183E-17,3.7));
#34670=CARTESIAN_POINT('Ctrl Pts',(-0.126614009842867,6.71750503076223E-5,
3.90565803263806));
#34671=CARTESIAN_POINT('Ctrl Pts',(-0.126638949568151,0.00394272317787337,
3.90541324973226));
#34672=CARTESIAN_POINT('Ctrl Pts',(-0.126476435154099,0.00781615144459198,
3.90516846682647));
#34673=CARTESIAN_POINT('Ctrl Pts',(-0.126119637661472,0.0116715998582211,
3.90492368392067));
#34674=CARTESIAN_POINT('Ctrl Pts',(-0.122261990910541,0.0533561922490439,
3.90227712389504));
#34675=CARTESIAN_POINT('Ctrl Pts',(-0.0956933418361204,0.0929390036289487,
3.89963056386942));
#34676=CARTESIAN_POINT('Ctrl Pts',(-0.0585765319889427,0.112299495998321,
3.89698400384379));
#34677=CARTESIAN_POINT('Ctrl Pts',(-0.0214597221417651,0.131659988367694,
3.89433744381817));
#34678=CARTESIAN_POINT('Ctrl Pts',(0.0262052484781696,0.130798161726534,
3.89169088379254));
#34679=CARTESIAN_POINT('Ctrl Pts',(0.0625979063415064,0.110108538679153,
3.88904432376692));
#34680=CARTESIAN_POINT('Ctrl Pts',(0.0989905642048431,0.089418915631772,
3.88639776374129));
#34681=CARTESIAN_POINT('Ctrl Pts',(0.124110909311582,0.04890149617817,3.88375120371567));
#34682=CARTESIAN_POINT('Ctrl Pts',(0.12645912901712,0.0071047004378325,
3.88110464369004));
#34683=CARTESIAN_POINT('Ctrl Pts',(0.128807348722658,-0.0346920953025048,
3.87845808366442));
#34684=CARTESIAN_POINT('Ctrl Pts',(0.108383443026996,-0.0777682673295779,
3.87581152363879));
#34685=CARTESIAN_POINT('Ctrl Pts',(0.0745372459479278,-0.102404036849921,
3.87316496361316));
#34686=CARTESIAN_POINT('Ctrl Pts',(0.0406910488688595,-0.127039806370264,
3.87051840358754));
#34687=CARTESIAN_POINT('Ctrl Pts',(-0.00657743959361464,-0.133235173383876,
3.86787184356191));
#34688=CARTESIAN_POINT('Ctrl Pts',(-0.0456292438338329,-0.118153967704968,
3.86522528353629));
#34689=CARTESIAN_POINT('Ctrl Pts',(-0.0846810480740508,-0.10307276202606,
3.86257872351066));
#34690=CARTESIAN_POINT('Ctrl Pts',(-0.115516168092013,-0.0667149836546316,
3.85993216348504));
#34691=CARTESIAN_POINT('Ctrl Pts',(-0.124018635887212,-0.0257248110583692,
3.85728560345941));
#34692=CARTESIAN_POINT('Ctrl Pts',(-0.125761573683066,-0.0173221539948553,
3.85674307985229));
#34693=CARTESIAN_POINT('Ctrl Pts',(-0.126566055107683,-0.00872483577640936,
3.85620055624518));
#34694=CARTESIAN_POINT('Ctrl Pts',(-0.126486618721746,-0.000112766438119152,
3.85565803263806));
#34695=CARTESIAN_POINT('Ctrl Pts',(-0.126249985800877,-2.99474503126992E-5,
3.86934196736194));
#34696=CARTESIAN_POINT('Ctrl Pts',(-0.126290782696275,-0.01929242997697,
3.87054968449796));
#34697=CARTESIAN_POINT('Ctrl Pts',(-0.12215616704665,-0.0385383011374065,
3.87175740163397));
#34698=CARTESIAN_POINT('Ctrl Pts',(-0.113755815955893,-0.0556956374040618,
3.87296511876998));
#34699=CARTESIAN_POINT('Ctrl Pts',(-0.0953475043280787,-0.0932937793492606,
3.87561167879561));
#34700=CARTESIAN_POINT('Ctrl Pts',(-0.0564546177286578,-0.120862525378353,
3.87825823882124));
#34701=CARTESIAN_POINT('Ctrl Pts',(-0.0148818774258165,-0.125781231309797,
3.88090479884686));
#34702=CARTESIAN_POINT('Ctrl Pts',(0.0266908628770249,-0.13069993724124,
3.88355135887249));
#34703=CARTESIAN_POINT('Ctrl Pts',(0.0709434568832867,-0.112968603075036,
3.88619791889811));
#34704=CARTESIAN_POINT('Ctrl Pts',(0.0976175698612337,-0.0807044039779288,
3.88884447892374));
#34705=CARTESIAN_POINT('Ctrl Pts',(0.124291682839181,-0.0484402048808214,
3.89149103894936));
#34706=CARTESIAN_POINT('Ctrl Pts',(0.133387314788813,-0.00164314085281106,
3.89413759897499));
#34707=CARTESIAN_POINT('Ctrl Pts',(0.120740589231085,0.0382635693618544,
3.89678415900061));
#34708=CARTESIAN_POINT('Ctrl Pts',(0.108093863673357,0.0781702795765198,
3.89943071902624));
#34709=CARTESIAN_POINT('Ctrl Pts',(0.0737047806082696,0.11118663597784,
3.90207727905187));
#34710=CARTESIAN_POINT('Ctrl Pts',(0.0333162705051194,0.122198232868137,
3.90472383907749));
#34711=CARTESIAN_POINT('Ctrl Pts',(-0.00707223959803082,0.133209829758434,
3.90737039910312));
#34712=CARTESIAN_POINT('Ctrl Pts',(-0.0534601767392434,0.122216667137707,
3.91001695912874));
#34713=CARTESIAN_POINT('Ctrl Pts',(-0.0846116689345932,0.0942510810621984,
3.91266351915437));
#34714=CARTESIAN_POINT('Ctrl Pts',(-0.110814692885301,0.0707278765512593,
3.91488966855689));
#34715=CARTESIAN_POINT('Ctrl Pts',(-0.126237468513852,0.0351961661111841,
3.91711581795942));
#34716=CARTESIAN_POINT('Ctrl Pts',(-0.126543984365092,-0.000100563349596846,
3.91934196736194));
#34717=CARTESIAN_POINT('Origin',(0.,0.,3.7));
#34718=CARTESIAN_POINT('',(-0.126567406925801,8.9117089303592E-5,3.96934196736194));
#34719=CARTESIAN_POINT('',(-0.126283770505697,7.06948412972308E-5,3.95565803263806));
#34720=CARTESIAN_POINT('',(-0.12645,1.54856587752183E-17,3.7));
#34721=CARTESIAN_POINT('',(0.0958116152722338,0.0825211298936549,4.));
#34722=CARTESIAN_POINT('Ctrl Pts',(-0.126567406925801,8.9117089303592E-5,
3.96934196736194));
#34723=CARTESIAN_POINT('Ctrl Pts',(-0.126271512495954,-0.03602989561222,
3.97162163149775));
#34724=CARTESIAN_POINT('Ctrl Pts',(-0.11000667585855,-0.0723734458913716,
3.97390129563356));
#34725=CARTESIAN_POINT('Ctrl Pts',(-0.0826932529987204,-0.0959262598695684,
3.97618095976937));
#34726=CARTESIAN_POINT('Ctrl Pts',(-0.0509839270641226,-0.123269733404333,
3.978827519795));
#34727=CARTESIAN_POINT('Ctrl Pts',(-0.0043834430999392,-0.133373998977298,
3.98147407982063));
#34728=CARTESIAN_POINT('Ctrl Pts',(0.0357753280219188,-0.121524403040669,
3.98412063984625));
#34729=CARTESIAN_POINT('Ctrl Pts',(0.0759340991437768,-0.109674807104039,
3.98676719987188));
#34730=CARTESIAN_POINT('Ctrl Pts',(0.109651157423309,-0.0758713496578151,
3.9894137598975));
#34731=CARTESIAN_POINT('Ctrl Pts',(0.121481684447537,-0.0357885393155276,
3.99206031992312));
#34732=CARTESIAN_POINT('Ctrl Pts',(0.133312211471764,0.00429427102675994,
3.99470687994875));
#34733=CARTESIAN_POINT('Ctrl Pts',(0.123256207240687,0.0506564342651108,
3.99735343997437));
#34734=CARTESIAN_POINT('Ctrl Pts',(0.095811615272233,0.0825211298936557,
4.));
#34735=CARTESIAN_POINT('',(-0.0959939867336434,0.082660026050108,4.));
#34736=CARTESIAN_POINT('Origin',(0.,0.,4.));
#34737=CARTESIAN_POINT('Ctrl Pts',(-0.095994151316856,0.0826601513985344,
4.));
#34738=CARTESIAN_POINT('Ctrl Pts',(-0.0693049200029063,0.113544200686508,
3.9974200549221));
#34739=CARTESIAN_POINT('Ctrl Pts',(-0.0262885035315151,0.130447365396717,
3.9948401098442));
#34740=CARTESIAN_POINT('Ctrl Pts',(0.0142676559974625,0.125842964228272,
3.9922601647663));
#34741=CARTESIAN_POINT('Ctrl Pts',(0.0558709876039151,0.121119676054917,
3.98961360474068));
#34742=CARTESIAN_POINT('Ctrl Pts',(0.0948853729157606,0.0937638197023474,
3.98696704471505));
#34743=CARTESIAN_POINT('Ctrl Pts',(0.113475682659087,0.0562620533584955,
3.98432048468943));
#34744=CARTESIAN_POINT('Ctrl Pts',(0.132065992402412,0.0187602870146438,
3.9816739246638));
#34745=CARTESIAN_POINT('Ctrl Pts',(0.130232226577219,-0.0288873893204904,
3.97902736463818));
#34746=CARTESIAN_POINT('Ctrl Pts',(0.108800980591427,-0.0648498109281795,
3.97638080461255));
#34747=CARTESIAN_POINT('Ctrl Pts',(0.0873697346056348,-0.100812232535869,
3.97373424458693));
#34748=CARTESIAN_POINT('Ctrl Pts',(0.046341008459244,-0.125089399416112,
3.9710876845613));
#34749=CARTESIAN_POINT('Ctrl Pts',(0.00450388209284308,-0.126577017215687,
3.96844112453568));
#34750=CARTESIAN_POINT('Ctrl Pts',(-0.0373332442735578,-0.128064635015261,
3.96579456451005));
#34751=CARTESIAN_POINT('Ctrl Pts',(-0.0799787708599689,-0.106762703734165,
3.96314800448442));
#34752=CARTESIAN_POINT('Ctrl Pts',(-0.103913438592044,-0.0724181315163075,
3.9605014444588));
#34753=CARTESIAN_POINT('Ctrl Pts',(-0.118514209844363,-0.0514670471592998,
3.95888697385188));
#34754=CARTESIAN_POINT('Ctrl Pts',(-0.126152075437054,-0.0256623813017284,
3.95727250324497));
#34755=CARTESIAN_POINT('Ctrl Pts',(-0.126283770505697,7.06948412972308E-5,
3.95565803263806));
#34756=CARTESIAN_POINT('Origin',(0.,0.,4.11042117235887));
#34757=CARTESIAN_POINT('',(-0.154553716617854,1.07385516829317E-5,3.53957882764113));
#34758=CARTESIAN_POINT('',(-0.154050307343621,3.81371511608408E-5,3.53542117235887));
#34759=CARTESIAN_POINT('',(-0.1543,7.47606542906876E-15,4.11042117235887));
#34760=CARTESIAN_POINT('',(0.0398513841857357,-0.149064942821848,3.5));
#34761=CARTESIAN_POINT('Ctrl Pts',(-0.154050307343621,3.81371511608431E-5,
3.53542117235887));
#34762=CARTESIAN_POINT('Ctrl Pts',(-0.154093326879583,0.0238011172149125,
3.53420035500841));
#34763=CARTESIAN_POINT('Ctrl Pts',(-0.137743852801688,0.0990167675561842,
3.53033297763233));
#34764=CARTESIAN_POINT('Ctrl Pts',(-0.0205691901156568,0.181176596665036,
3.52381904023063));
#34765=CARTESIAN_POINT('Ctrl Pts',(0.141207069227503,0.115615351338242,
3.51587936015375));
#34766=CARTESIAN_POINT('Ctrl Pts',(0.173454096992073,-0.0561631599472297,
3.50793968007688));
#34767=CARTESIAN_POINT('Ctrl Pts',(0.089426887306191,-0.135811307301286,
3.50264656002563));
#34768=CARTESIAN_POINT('Ctrl Pts',(0.0398513841857336,-0.149064942821849,
3.5));
#34769=CARTESIAN_POINT('',(-0.0398513841857265,-0.149064942821851,3.5));
#34770=CARTESIAN_POINT('Origin',(0.,0.,3.5));
#34771=CARTESIAN_POINT('Ctrl Pts',(-0.154553716617854,1.07385516829459E-5,
3.53957882764113));
#34772=CARTESIAN_POINT('Ctrl Pts',(-0.154554183576509,0.000527195138975443,
3.53955207027449));
#34773=CARTESIAN_POINT('Ctrl Pts',(-0.154317915988944,0.0521256879879336,
3.53687875288222));
#34774=CARTESIAN_POINT('Ctrl Pts',(-0.0973408901199132,0.154229940417525,
3.53155887546432));
#34775=CARTESIAN_POINT('Ctrl Pts',(0.0768181056158631,0.16543527210962,
3.52361919538745));
#34776=CARTESIAN_POINT('Ctrl Pts',(0.180643771975638,0.0251157687415861,
3.51567951531057));
#34777=CARTESIAN_POINT('Ctrl Pts',(0.119593430082514,-0.13672026231454,
3.50780645018142));
#34778=CARTESIAN_POINT('Ctrl Pts',(0.00819996357198913,-0.162114976519676,
3.5025799450779));
#34779=CARTESIAN_POINT('Ctrl Pts',(-0.0399398165374138,-0.14933059314829,
3.5));
#34780=CARTESIAN_POINT('Origin',(0.,0.,4.11042117235887));
#34781=CARTESIAN_POINT('',(-0.15419083216807,0.000129561635314926,3.58957882764113));
#34782=CARTESIAN_POINT('',(-0.154288256028425,-0.000141223516069758,3.58542117235887));
#34783=CARTESIAN_POINT('',(-0.1543,7.47606542906876E-15,4.11042117235887));
#34784=CARTESIAN_POINT('Ctrl Pts',(-0.154288256028425,-0.000141223516069763,
3.58542117235887));
#34785=CARTESIAN_POINT('Ctrl Pts',(-0.153932746614783,0.0387932487575316,
3.5834130484955));
#34786=CARTESIAN_POINT('Ctrl Pts',(-0.119227247372343,0.129604846059009,
3.57875836460651));
#34787=CARTESIAN_POINT('Ctrl Pts',(0.0333654249967142,0.179306991453011,
3.57145712069188));
#34788=CARTESIAN_POINT('Ctrl Pts',(0.16875469474836,0.0691889591605158,
3.56351744061501));
#34789=CARTESIAN_POINT('Ctrl Pts',(0.149631713131164,-0.104283094234219,
3.55557776053813));
#34790=CARTESIAN_POINT('Ctrl Pts',(-0.00648228852693025,-0.182263845309582,
3.54763808046125));
#34791=CARTESIAN_POINT('Ctrl Pts',(-0.133583343879226,-0.107056676726779,
3.54091921773484));
#34792=CARTESIAN_POINT('Ctrl Pts',(-0.154000066586259,-0.0277136758071254,
3.53684691503404));
#34793=CARTESIAN_POINT('Ctrl Pts',(-0.154050307343621,3.81371511608431E-5,
3.53542117235887));
#34794=CARTESIAN_POINT('Ctrl Pts',(-0.15419083216807,0.000129561635314916,
3.58957882764113));
#34795=CARTESIAN_POINT('Ctrl Pts',(-0.154316540000352,0.0159383321389732,
3.58876476376157));
#34796=CARTESIAN_POINT('Ctrl Pts',(-0.144808574808872,0.0829945710278969,
3.58530413985639));
#34797=CARTESIAN_POINT('Ctrl Pts',(-0.0479747871584019,0.175962994372803,
3.57919695592558));
#34798=CARTESIAN_POINT('Ctrl Pts',(0.121839171429706,0.13571993663382,3.5712572758487));
#34799=CARTESIAN_POINT('Ctrl Pts',(0.180099946935509,-0.0287862221383337,
3.56331759577183));
#34800=CARTESIAN_POINT('Ctrl Pts',(0.0734653204375665,-0.166934393666355,
3.55537791569495));
#34801=CARTESIAN_POINT('Ctrl Pts',(-0.0998464626320651,-0.152294592499083,
3.54746499298472));
#34802=CARTESIAN_POINT('Ctrl Pts',(-0.154507996889821,-0.0505553114913108,
3.54219863030011));
#34803=CARTESIAN_POINT('Ctrl Pts',(-0.154553716617854,1.07385516829459E-5,
3.53957882764113));
#34804=CARTESIAN_POINT('Origin',(0.,0.,4.11042117235887));
#34805=CARTESIAN_POINT('',(-0.154093198061062,-8.33060061860361E-5,3.63957882764113));
#34806=CARTESIAN_POINT('',(-0.154532949196129,5.22176212347235E-5,3.63542117235887));
#34807=CARTESIAN_POINT('',(-0.1543,7.47606542906876E-15,4.11042117235887));
#34808=CARTESIAN_POINT('Ctrl Pts',(-0.154532949196129,5.22176212347084E-5,
3.63542117235887));
#34809=CARTESIAN_POINT('Ctrl Pts',(-0.154545584588578,0.00292672178698735,
3.63527230200821));
#34810=CARTESIAN_POINT('Ctrl Pts',(-0.153169988902963,0.0568907246896308,
3.63247687163192));
#34811=CARTESIAN_POINT('Ctrl Pts',(-0.0901397813258339,0.158554191001936,
3.62703488123002));
#34812=CARTESIAN_POINT('Ctrl Pts',(0.0843490755327352,0.161709110561297,
3.61909520115314));
#34813=CARTESIAN_POINT('Ctrl Pts',(0.181609876119891,0.0168069020193158,
3.61115552107626));
#34814=CARTESIAN_POINT('Ctrl Pts',(0.11259272547993,-0.14348343554309,3.60321584099938));
#34815=CARTESIAN_POINT('Ctrl Pts',(-0.0595116136917225,-0.1724033835878,
3.59527616092251));
#34816=CARTESIAN_POINT('Ctrl Pts',(-0.147380741016298,-0.0760839947500021,
3.58934460470901));
#34817=CARTESIAN_POINT('Ctrl Pts',(-0.154401281957667,-0.0125195312047306,
3.58605960852113));
#34818=CARTESIAN_POINT('Ctrl Pts',(-0.154288256028425,-0.000141223516069763,
3.58542117235887));
#34819=CARTESIAN_POINT('Ctrl Pts',(-0.154093198061063,-8.33060061860274E-5,
3.63957882764113));
#34820=CARTESIAN_POINT('Ctrl Pts',(-0.153940587938977,0.0310641981069166,
3.63797745724865));
#34821=CARTESIAN_POINT('Ctrl Pts',(-0.129646233104354,0.113907608400038,
3.63372952683056));
#34822=CARTESIAN_POINT('Ctrl Pts',(0.00558664719359638,0.182300288895857,
3.62683503638684));
#34823=CARTESIAN_POINT('Ctrl Pts',(0.156205528517827,0.094151159125646,
3.61889535630996));
#34824=CARTESIAN_POINT('Ctrl Pts',(0.163806179027695,-0.0802006497663837,
3.61095567623308));
#34825=CARTESIAN_POINT('Ctrl Pts',(0.0214296163208854,-0.181122531330724,
3.60301599615621));
#34826=CARTESIAN_POINT('Ctrl Pts',(-0.123957687612568,-0.122868073634794,
3.59589037995889));
#34827=CARTESIAN_POINT('Ctrl Pts',(-0.1539078579151,-0.0354567255707862,
3.5914113237872));
#34828=CARTESIAN_POINT('Ctrl Pts',(-0.15419083216807,0.000129561635314916,
3.58957882764113));
#34829=CARTESIAN_POINT('Origin',(0.,0.,4.11042117235887));
#34830=CARTESIAN_POINT('',(-0.154494739391599,-8.56666717596894E-5,3.68957882764113));
#34831=CARTESIAN_POINT('',(-0.15413359010754,0.000108847378321225,3.68542117235887));
#34832=CARTESIAN_POINT('',(-0.1543,7.47606542906876E-15,4.11042117235887));
#34833=CARTESIAN_POINT('Ctrl Pts',(-0.15413359010754,0.00010884737832121,
3.68542117235887));
#34834=CARTESIAN_POINT('Ctrl Pts',(-0.154252061492927,0.0183060191525707,
3.6844849954953));
#34835=CARTESIAN_POINT('Ctrl Pts',(-0.142855501009428,0.0878027720491901,
3.6809022586061));
#34836=CARTESIAN_POINT('Ctrl Pts',(-0.039826269011209,0.177984489264188,
3.67467296169127));
#34837=CARTESIAN_POINT('Ctrl Pts',(0.127955809817362,0.129968921992697,
3.66673328161439));
#34838=CARTESIAN_POINT('Ctrl Pts',(0.178584458888466,-0.0370432344610292,
3.65879360153752));
#34839=CARTESIAN_POINT('Ctrl Pts',(0.0657052360091523,-0.170139449612234,
3.65085392146064));
#34840=CARTESIAN_POINT('Ctrl Pts',(-0.104087723049408,-0.147885095147454,
3.64306311173443));
#34841=CARTESIAN_POINT('Ctrl Pts',(-0.154320957425313,-0.0481751113503961,
3.63791886203384));
#34842=CARTESIAN_POINT('Ctrl Pts',(-0.154532949196129,5.22176212347084E-5,
3.63542117235887));
#34843=CARTESIAN_POINT('Ctrl Pts',(-0.154494739391599,-8.56666717596998E-5,
3.68957882764113));
#34844=CARTESIAN_POINT('Ctrl Pts',(-0.15418701910941,0.0460669561753479,
3.68719015073574));
#34845=CARTESIAN_POINT('Ctrl Pts',(-0.107714707332757,0.143892491682726,
3.68215491380472));
#34846=CARTESIAN_POINT('Ctrl Pts',(0.0586595287281965,0.172695299861449,
3.67447311684809));
#34847=CARTESIAN_POINT('Ctrl Pts',(0.176911729524118,0.0443491475303153,
3.66653343677121));
#34848=CARTESIAN_POINT('Ctrl Pts',(0.133187572742707,-0.124602076359984,
3.65859375669434));
#34849=CARTESIAN_POINT('Ctrl Pts',(-0.0324800977009374,-0.179470471240069,
3.65065407661746));
#34850=CARTESIAN_POINT('Ctrl Pts',(-0.140993802389242,-0.0920951181032393,
3.64431576693306));
#34851=CARTESIAN_POINT('Ctrl Pts',(-0.154192804322217,-0.0204127991394723,
3.64062401727428));
#34852=CARTESIAN_POINT('Ctrl Pts',(-0.154093198061063,-8.33060061860274E-5,
3.63957882764113));
#34853=CARTESIAN_POINT('Origin',(0.,0.,4.11042117235887));
#34854=CARTESIAN_POINT('',(-0.154352374546534,0.000136543067356262,3.73957882764113));
#34855=CARTESIAN_POINT('',(-0.154139174508622,-0.000111501026995055,3.73542117235887));
#34856=CARTESIAN_POINT('',(-0.1543,7.47606542906876E-15,4.11042117235887));
#34857=CARTESIAN_POINT('Ctrl Pts',(-0.154139174508622,-0.000111501026995059,
3.73542117235887));
#34858=CARTESIAN_POINT('Ctrl Pts',(-0.153915233552703,0.0333860868580806,
3.73369768898238));
#34859=CARTESIAN_POINT('Ctrl Pts',(-0.1267153517394,0.118653316414882,3.72932764558026));
#34860=CARTESIAN_POINT('Ctrl Pts',(0.0139700521550768,0.18185006934563,
3.72231104215253));
#34861=CARTESIAN_POINT('Ctrl Pts',(0.160372810275332,0.0868629483698537,
3.71437136207565));
#34862=CARTESIAN_POINT('Ctrl Pts',(0.15994186929589,-0.087653913339944,
3.70643168199877));
#34863=CARTESIAN_POINT('Ctrl Pts',(0.013071788942189,-0.181916844788939,
3.6984920019219));
#34864=CARTESIAN_POINT('Ctrl Pts',(-0.127037714877433,-0.11814535336758,
3.6914884987086));
#34865=CARTESIAN_POINT('Ctrl Pts',(-0.153917144400928,-0.0331371528280101,
3.68713155552092));
#34866=CARTESIAN_POINT('Ctrl Pts',(-0.15413359010754,0.00010884737832121,
3.68542117235887));
#34867=CARTESIAN_POINT('Ctrl Pts',(-0.154352374546534,0.000136543067356257,
3.73957882764113));
#34868=CARTESIAN_POINT('Ctrl Pts',(-0.154446737273245,0.0103903099163322,
3.73904940424845));
#34869=CARTESIAN_POINT('Ctrl Pts',(-0.148841316561083,0.0717994892151511,
3.73587342083015));
#34870=CARTESIAN_POINT('Ctrl Pts',(-0.0665446905722607,0.169812870767156,
3.73005087738622));
#34871=CARTESIAN_POINT('Ctrl Pts',(0.106602640202898,0.147988121222216,
3.72211119730934));
#34872=CARTESIAN_POINT('Ctrl Pts',(0.182147017152552,-0.0093311876933208,
3.71417151723247));
#34873=CARTESIAN_POINT('Ctrl Pts',(0.0909217261957518,-0.158107073301583,
3.70623183715559));
#34874=CARTESIAN_POINT('Ctrl Pts',(-0.0835494302172658,-0.162123717048593,
3.69829215707872));
#34875=CARTESIAN_POINT('Ctrl Pts',(-0.152048491522357,-0.0611528114853893,
3.69274115390723));
#34876=CARTESIAN_POINT('Ctrl Pts',(-0.154527961074428,-0.00506833400535766,
3.68983671076137));
#34877=CARTESIAN_POINT('Ctrl Pts',(-0.154494739391599,-8.56666717596998E-5,
3.68957882764113));
#34878=CARTESIAN_POINT('Origin',(0.,0.,4.11042117235887));
#34879=CARTESIAN_POINT('',(-0.154047977067031,2.09413777367551E-6,3.78957882764113));
#34880=CARTESIAN_POINT('',(-0.154536408180499,-4.7848165513455E-5,3.78542117235887));
#34881=CARTESIAN_POINT('',(-0.1543,7.47606542906876E-15,4.11042117235887));
#34882=CARTESIAN_POINT('Ctrl Pts',(-0.154536408180499,-4.78481655134459E-5,
3.78542117235887));
#34883=CARTESIAN_POINT('Ctrl Pts',(-0.154339106087067,0.0484295369338371,
3.78291038246947));
#34884=CARTESIAN_POINT('Ctrl Pts',(-0.103641790719782,0.148361335894058,
3.77775303255443));
#34885=CARTESIAN_POINT('Ctrl Pts',(0.0665446937287967,0.169812878822259,
3.76994912261378));
#34886=CARTESIAN_POINT('Ctrl Pts',(0.178765223990991,0.0361608181406009,
3.7620094425369));
#34887=CARTESIAN_POINT('Ctrl Pts',(0.127312379282745,-0.130599265535886,
3.75406976246003));
#34888=CARTESIAN_POINT('Ctrl Pts',(-0.0407047855299705,-0.177785630781348,
3.74613008238315));
#34889=CARTESIAN_POINT('Ctrl Pts',(-0.143071654254016,-0.0872869087240706,
3.73991388568277));
#34890=CARTESIAN_POINT('Ctrl Pts',(-0.154259114549828,-0.0180524000230757,
3.73634424900801));
#34891=CARTESIAN_POINT('Ctrl Pts',(-0.154139174508622,-0.000111501026995059,
3.73542117235887));
#34892=CARTESIAN_POINT('Ctrl Pts',(-0.154047977067031,2.09413777367898E-6,
3.78957882764113));
#34893=CARTESIAN_POINT('Ctrl Pts',(-0.154051078605937,0.0256319813134887,
3.78826209773554));
#34894=CARTESIAN_POINT('Ctrl Pts',(-0.135851564244815,0.102772493157479,
3.78429880780432));
#34895=CARTESIAN_POINT('Ctrl Pts',(-0.013970051492431,0.181850060719556,
3.77768895784748));
#34896=CARTESIAN_POINT('Ctrl Pts',(0.145223361235896,0.110339395832533,
3.7697492777706));
#34897=CARTESIAN_POINT('Ctrl Pts',(0.171453565975463,-0.0621955113766863,
3.76180959769372));
#34898=CARTESIAN_POINT('Ctrl Pts',(0.0407047835991549,-0.177785622348059,
3.75386991761685));
#34899=CARTESIAN_POINT('Ctrl Pts',(-0.11610887230377,-0.133745678862782,
3.74645966093265));
#34900=CARTESIAN_POINT('Ctrl Pts',(-0.153975022906486,-0.0408677376689339,
3.74169596427408));
#34901=CARTESIAN_POINT('Ctrl Pts',(-0.154352374546534,0.000136543067356257,
3.73957882764113));
#34902=CARTESIAN_POINT('Origin',(0.,0.,4.11042117235887));
#34903=CARTESIAN_POINT('',(-0.154344683817836,-0.000137602699895489,3.83957882764113));
#34904=CARTESIAN_POINT('',(-0.154280621254558,0.000141160201694546,3.83542117235887));
#34905=CARTESIAN_POINT('',(-0.1543,7.47606542906876E-15,4.11042117235887));
#34906=CARTESIAN_POINT('Ctrl Pts',(-0.154280621254558,0.000141160201694572,
3.83542117235887));
#34907=CARTESIAN_POINT('Ctrl Pts',(-0.154395390544122,0.0127750301081681,
3.83476963598218));
#34908=CARTESIAN_POINT('Ctrl Pts',(-0.147198204620896,0.0765990159781269,
3.83147153957986));
#34909=CARTESIAN_POINT('Ctrl Pts',(-0.0586595315107243,0.172695308053416,
3.82552688315191));
#34910=CARTESIAN_POINT('Ctrl Pts',(0.113300008356683,0.142925568707939,
3.81758720307504));
#34911=CARTESIAN_POINT('Ctrl Pts',(0.181524636378177,-0.0177035721096275,
3.80964752299816));
#34912=CARTESIAN_POINT('Ctrl Pts',(0.0835494341804624,-0.162123724738966,
3.80170784292129));
#34913=CARTESIAN_POINT('Ctrl Pts',(-0.0909217305086156,-0.158107080801413,
3.7937681628444));
#34914=CARTESIAN_POINT('Ctrl Pts',(-0.15329856504372,-0.056379054482583,
3.78833927265694));
#34915=CARTESIAN_POINT('Ctrl Pts',(-0.154547077226211,-0.00266924679639216,
3.78555694249509));
#34916=CARTESIAN_POINT('Ctrl Pts',(-0.154536408180499,-4.78481655134459E-5,
3.78542117235887));
#34917=CARTESIAN_POINT('Ctrl Pts',(-0.154344683817836,-0.000137602699895493,
3.83957882764113));
#34918=CARTESIAN_POINT('Ctrl Pts',(-0.153968758841032,0.0406181785207979,
3.83747479122262));
#34919=CARTESIAN_POINT('Ctrl Pts',(-0.11649114353226,0.133249851238064,
3.83272419477849));
#34920=CARTESIAN_POINT('Ctrl Pts',(0.039826267121788,0.177984480821945,
3.82532703830873));
#34921=CARTESIAN_POINT('Ctrl Pts',(0.171144313607041,0.063041501012073,
3.81738735823185));
#34922=CARTESIAN_POINT('Ctrl Pts',(0.145766517224248,-0.109620843643728,
3.80944767815498));
#34923=CARTESIAN_POINT('Ctrl Pts',(-0.0130717883220708,-0.181916836159762,
3.8015079980781));
#34924=CARTESIAN_POINT('Ctrl Pts',(-0.135584681571728,-0.103286631626578,
3.79488504790682));
#34925=CARTESIAN_POINT('Ctrl Pts',(-0.154044844670753,-0.0258827861209538,
3.79090865776116));
#34926=CARTESIAN_POINT('Ctrl Pts',(-0.154047977067031,2.09413777367898E-6,
3.78957882764113));
#34927=CARTESIAN_POINT('Origin',(0.,0.,4.11042117235887));
#34928=CARTESIAN_POINT('',(-0.154500132216325,8.19700297638587E-5,3.88957882764113));
#34929=CARTESIAN_POINT('',(-0.154055933642351,-3.65432311820964E-5,3.88542117235887));
#34930=CARTESIAN_POINT('',(-0.1543,7.47606542906876E-15,4.11042117235887));
#34931=CARTESIAN_POINT('Ctrl Pts',(-0.154055933642351,-3.6543231182122E-5,
3.88542117235887));
#34932=CARTESIAN_POINT('Ctrl Pts',(-0.15399662440304,0.0279666460980613,
3.88398232946926));
#34933=CARTESIAN_POINT('Ctrl Pts',(-0.133294661580101,0.10755966601202,
3.87989692655402));
#34934=CARTESIAN_POINT('Ctrl Pts',(-0.005586647457645,0.182300297549597,
3.87316496361317));
#34935=CARTESIAN_POINT('Ctrl Pts',(0.150147248343024,0.103539432915148,
3.86522528353629));
#34936=CARTESIAN_POINT('Ctrl Pts',(0.168409737102627,-0.0700197873807462,
3.85728560345941));
#34937=CARTESIAN_POINT('Ctrl Pts',(0.0324800992415292,-0.179470479754251,
3.84934592338254));
#34938=CARTESIAN_POINT('Ctrl Pts',(-0.1195927593937,-0.129104626018084,
3.84205777968236));
#34939=CARTESIAN_POINT('Ctrl Pts',(-0.153929194296616,-0.0385441229881096,
3.8374161960078));
#34940=CARTESIAN_POINT('Ctrl Pts',(-0.154280621254558,0.000141160201694572,
3.83542117235887));
#34941=CARTESIAN_POINT('Ctrl Pts',(-0.154500132216325,8.19700297638379E-5,
3.88957882764113));
#34942=CARTESIAN_POINT('Ctrl Pts',(-0.1545305647953,0.00481108885999716,
3.88933404473533));
#34943=CARTESIAN_POINT('Ctrl Pts',(-0.152188184006249,0.0606402533846132,
3.88644270180391));
#34944=CARTESIAN_POINT('Ctrl Pts',(-0.0843490715154628,0.161709102853824,
3.88090479884686));
#34945=CARTESIAN_POINT('Ctrl Pts',(0.0901397770410241,0.158554183500776,
3.87296511876998));
#34946=CARTESIAN_POINT('Ctrl Pts',(0.182098715355847,0.0102306290122647,
3.86502543869311));
#34947=CARTESIAN_POINT('Ctrl Pts',(0.107332199369115,-0.147459841777235,
3.85708575861623));
#34948=CARTESIAN_POINT('Ctrl Pts',(-0.0657052328909015,-0.17013944154474,
3.84914607853936));
#34949=CARTESIAN_POINT('Ctrl Pts',(-0.148671156397415,-0.0723140833987834,
3.84331043488099));
#34950=CARTESIAN_POINT('Ctrl Pts',(-0.154441615683002,-0.0106464385947012,
3.84012135124824));
#34951=CARTESIAN_POINT('Ctrl Pts',(-0.154344683817836,-0.000137602699895493,
3.83957882764113));
#34952=CARTESIAN_POINT('Origin',(0.,0.,4.11042117235887));
#34953=CARTESIAN_POINT('',(-0.154097159264761,8.62650376686758E-5,3.93957882764113));
#34954=CARTESIAN_POINT('',(-0.154414683966261,-0.000122711940234539,3.93542117235887));
#34955=CARTESIAN_POINT('',(-0.1543,7.47606542906876E-15,4.11042117235887));
#34956=CARTESIAN_POINT('Ctrl Pts',(-0.154414683966261,-0.00012271194023455,
3.93542117235887));
#34957=CARTESIAN_POINT('Ctrl Pts',(-0.15404065948349,0.0429479512135688,
3.93319502295635));
#34958=CARTESIAN_POINT('Ctrl Pts',(-0.11284743018063,0.1378508358131,3.9283223135282));
#34959=CARTESIAN_POINT('Ctrl Pts',(0.0479747894892283,0.175963002958517,
3.92080304407442));
#34960=CARTESIAN_POINT('Ctrl Pts',(0.173864125597012,0.0550988560374321,
3.91286336399754));
#34961=CARTESIAN_POINT('Ctrl Pts',(0.140567423109983,-0.116212816074597,
3.90492368392067));
#34962=CARTESIAN_POINT('Ctrl Pts',(-0.0214296173447312,-0.181122539961793,
3.89698400384379));
#34963=CARTESIAN_POINT('Ctrl Pts',(-0.138004452641611,-0.0984898965999405,
3.89048316665653));
#34964=CARTESIAN_POINT('Ctrl Pts',(-0.154105715856349,-0.0235414942304966,
3.88662888949489));
#34965=CARTESIAN_POINT('Ctrl Pts',(-0.154055933642351,-3.6543231182122E-5,
3.88542117235887));
#34966=CARTESIAN_POINT('Ctrl Pts',(-0.154097159264761,8.62650376686723E-5,
3.93957882764113));
#34967=CARTESIAN_POINT('Ctrl Pts',(-0.154199890802351,0.0201598980625174,
3.93854673822241));
#34968=CARTESIAN_POINT('Ctrl Pts',(-0.141224360537215,0.0915805799143205,
3.93486808877808));
#34969=CARTESIAN_POINT('Ctrl Pts',(-0.0333654229848094,0.179306981584077,
3.92854287930812));
#34970=CARTESIAN_POINT('Ctrl Pts',(0.132570265831228,0.125258780485074,
3.92060319923124));
#34971=CARTESIAN_POINT('Ctrl Pts',(0.17712875926901,-0.0434751369680033,
3.91266351915436));
#34972=CARTESIAN_POINT('Ctrl Pts',(0.059511610779771,-0.172403375181386,
3.90472383907749));
#34973=CARTESIAN_POINT('Ctrl Pts',(-0.107286687880009,-0.144375040164272,
3.89702894190641));
#34974=CARTESIAN_POINT('Ctrl Pts',(-0.154201531823291,-0.0463195111784584,
3.89198060476095));
#34975=CARTESIAN_POINT('Ctrl Pts',(-0.154500132216325,8.19700297638379E-5,
3.88957882764113));
#34976=CARTESIAN_POINT('Origin',(0.,0.,4.11042117235887));
#34977=CARTESIAN_POINT('',(-0.154145398954164,-0.00018319008806407,3.98957882764113));
#34978=CARTESIAN_POINT('',(-0.154443265232512,0.000108744696557919,3.98542117235887));
#34979=CARTESIAN_POINT('',(-0.1543,7.47606542906876E-15,4.11042117235887));
#34980=CARTESIAN_POINT('',(-0.0398513841857263,-0.149064942821851,4.));
#34981=CARTESIAN_POINT('Ctrl Pts',(-0.0398513841857263,-0.149064942821851,
4.));
#34982=CARTESIAN_POINT('Ctrl Pts',(-0.0894268873061843,-0.13581130730129,
3.99735343997437));
#34983=CARTESIAN_POINT('Ctrl Pts',(-0.144571567721208,-0.0835405737349159,
3.99387971585475));
#34984=CARTESIAN_POINT('Ctrl Pts',(-0.154267320225706,-0.0162511224334367,
3.99040599173513));
#34985=CARTESIAN_POINT('Ctrl Pts',(-0.154145398954164,-0.000183190088064077,
3.98957882764113));
#34986=CARTESIAN_POINT('',(0.0399397509085001,-0.149330346493117,4.));
#34987=CARTESIAN_POINT('Origin',(0.,0.,4.));
#34988=CARTESIAN_POINT('Ctrl Pts',(0.0399398308045223,-0.149330586455588,
4.));
#34989=CARTESIAN_POINT('Ctrl Pts',(-0.00819994193508078,-0.162114963086391,
3.9974200549221));
#34990=CARTESIAN_POINT('Ctrl Pts',(-0.111773735607764,-0.138502981643238,
3.99256044570839));
#34991=CARTESIAN_POINT('Ctrl Pts',(-0.154082201487749,-0.0439653055987776,
3.98770083649468));
#34992=CARTESIAN_POINT('Ctrl Pts',(-0.154443265232512,0.000108744696557906,
3.98542117235887));
#34993=CARTESIAN_POINT('Origin',(-1.70916393953233E-17,-6.81365885416763E-18,
3.5));
#34994=CARTESIAN_POINT('Ctrl Pts',(-0.0958116152722498,0.0825211298936362,
3.5));
#34995=CARTESIAN_POINT('Ctrl Pts',(-0.100695982673166,0.0779597798732974,
3.5));
#34996=CARTESIAN_POINT('Ctrl Pts',(-0.105169094336774,0.073000191113619,
3.5));
#34997=CARTESIAN_POINT('Ctrl Pts',(-0.109227190160158,0.0677117533966587,
3.5));
#34998=CARTESIAN_POINT('Ctrl Pts',(-0.111694873825402,0.0644959122887171,
3.5));
#34999=CARTESIAN_POINT('Ctrl Pts',(-0.114010184214277,0.0611562073506752,
3.5));
#35000=CARTESIAN_POINT('Ctrl Pts',(-0.116166807098829,0.0577125335531249,
3.5));
#35001=CARTESIAN_POINT('Ctrl Pts',(-0.121431726365849,0.0493055632589991,
3.5));
#35002=CARTESIAN_POINT('Ctrl Pts',(-0.12573464769667,0.0403151423737322,
3.5));
#35003=CARTESIAN_POINT('Ctrl Pts',(-0.129045466546674,0.0309386517006337,
3.5));
#35004=CARTESIAN_POINT('Ctrl Pts',(-0.130207164312345,0.0276486353154881,
3.5));
#35005=CARTESIAN_POINT('Ctrl Pts',(-0.131243087485824,0.0243197585947972,
3.5));
#35006=CARTESIAN_POINT('Ctrl Pts',(-0.132152263806834,0.0209620064696601,
3.5));
#35007=CARTESIAN_POINT('Ctrl Pts',(-0.134828933182204,0.0110765837240964,
3.5));
#35008=CARTESIAN_POINT('Ctrl Pts',(-0.136412178238084,0.000939292992310017,
3.5));
#35009=CARTESIAN_POINT('Ctrl Pts',(-0.136856372906323,-0.00925247465139327,
3.5));
#35010=CARTESIAN_POINT('Ctrl Pts',(-0.137021913483504,-0.0130506992112034,
3.5));
#35011=CARTESIAN_POINT('Ctrl Pts',(-0.137028726314264,-0.0168567537781713,
3.5));
#35012=CARTESIAN_POINT('Ctrl Pts',(-0.136872398016052,-0.0206609891299379,
3.5));
#35013=CARTESIAN_POINT('Ctrl Pts',(-0.136740582821431,-0.0238687002674301,
3.5));
#35014=CARTESIAN_POINT('Ctrl Pts',(-0.136493094718847,-0.0270653690856263,
3.5));
#35015=CARTESIAN_POINT('Ctrl Pts',(-0.13612917734588,-0.0302430275614766,
3.5));
#35016=CARTESIAN_POINT('Ctrl Pts',(-0.13576659429471,-0.0334090349888054,
3.5));
#35017=CARTESIAN_POINT('Ctrl Pts',(-0.135288410857674,-0.0365568188154616,
3.5));
#35018=CARTESIAN_POINT('Ctrl Pts',(-0.134693327673148,-0.0396806409761667,
3.5));
#35019=CARTESIAN_POINT('Ctrl Pts',(-0.133341599676801,-0.0467763848654778,
3.5));
#35020=CARTESIAN_POINT('Ctrl Pts',(-0.131387825400402,-0.0537485551880799,
3.5));
#35021=CARTESIAN_POINT('Ctrl Pts',(-0.128888271219693,-0.0605519919600177,
3.5));
#35022=CARTESIAN_POINT('Ctrl Pts',(-0.127520602506107,-0.0642745948504241,
3.5));
#35023=CARTESIAN_POINT('Ctrl Pts',(-0.125989250183059,-0.0679466858359917,
3.5));
#35024=CARTESIAN_POINT('Ctrl Pts',(-0.124301567034569,-0.0715605953668731,
3.5));
#35025=CARTESIAN_POINT('Ctrl Pts',(-0.123083413065749,-0.0741690815877246,
3.5));
#35026=CARTESIAN_POINT('Ctrl Pts',(-0.121784536276434,-0.0767452222753887,
3.5));
#35027=CARTESIAN_POINT('Ctrl Pts',(-0.120412533496435,-0.0792783080753084,
3.5));
#35028=CARTESIAN_POINT('Ctrl Pts',(-0.116240621079353,-0.0869807794232376,
3.5));
#35029=CARTESIAN_POINT('Ctrl Pts',(-0.111384900653015,-0.0943068033536031,
3.5));
#35030=CARTESIAN_POINT('Ctrl Pts',(-0.105936294580107,-0.101180758720708,
3.5));
#35031=CARTESIAN_POINT('Ctrl Pts',(-0.102498213514854,-0.105518237972245,
3.5));
#35032=CARTESIAN_POINT('Ctrl Pts',(-0.0988234872002696,-0.109675688132788,
3.5));
#35033=CARTESIAN_POINT('Ctrl Pts',(-0.0949300211352312,-0.113632240993693,
3.5));
#35034=CARTESIAN_POINT('Ctrl Pts',(-0.0916236146803262,-0.116992221972066,
3.5));
#35035=CARTESIAN_POINT('Ctrl Pts',(-0.0881545091528211,-0.120210812929281,
3.5));
#35036=CARTESIAN_POINT('Ctrl Pts',(-0.0845585132916744,-0.123253141705618,
3.5));
#35037=CARTESIAN_POINT('Ctrl Pts',(-0.0763242263006133,-0.13021961475866,
3.5));
#35038=CARTESIAN_POINT('Ctrl Pts',(-0.0674109291876633,-0.136284624413674,
3.5));
#35039=CARTESIAN_POINT('Ctrl Pts',(-0.0579550193346048,-0.141304740223277,
3.5));
#35040=CARTESIAN_POINT('Ctrl Pts',(-0.0532842084112166,-0.143784460538354,
3.5));
#35041=CARTESIAN_POINT('Ctrl Pts',(-0.0484803425336181,-0.146008805046434,
3.5));
#35042=CARTESIAN_POINT('Ctrl Pts',(-0.0435567265409999,-0.147956912059339,
3.5));
#35043=CARTESIAN_POINT('Ctrl Pts',(-0.042358096554505,-0.148431169086302,
3.5));
#35044=CARTESIAN_POINT('Ctrl Pts',(-0.0411523620931259,-0.148889040418797,
3.5));
#35045=CARTESIAN_POINT('Ctrl Pts',(-0.0399398165374117,-0.14933059314829,
3.5));
#35046=CARTESIAN_POINT('Ctrl Pts',(0.0398513841857336,-0.149064942821849,
3.5));
#35047=CARTESIAN_POINT('Ctrl Pts',(0.0462529496128914,-0.146725837162888,
3.5));
#35048=CARTESIAN_POINT('Ctrl Pts',(0.0524692076951892,-0.14393427563735,
3.5));
#35049=CARTESIAN_POINT('Ctrl Pts',(0.0584702623153416,-0.140728485236784,
3.5));
#35050=CARTESIAN_POINT('Ctrl Pts',(0.0631250229031883,-0.138241891170577,
3.5));
#35051=CARTESIAN_POINT('Ctrl Pts',(0.0676502468975603,-0.1355058910355,
3.5));
#35052=CARTESIAN_POINT('Ctrl Pts',(0.0720296458894365,-0.132535875720451,
3.5));
#35053=CARTESIAN_POINT('Ctrl Pts',(0.0754784967726087,-0.130196938354537,
3.5));
#35054=CARTESIAN_POINT('Ctrl Pts',(0.0788293975632557,-0.127717841671465,
3.5));
#35055=CARTESIAN_POINT('Ctrl Pts',(0.0820734025861846,-0.125108353169529,
3.5));
#35056=CARTESIAN_POINT('Ctrl Pts',(0.0878699486728443,-0.120445592089575,
3.5));
#35057=CARTESIAN_POINT('Ctrl Pts',(0.0933277488655726,-0.115365506062939,
3.5));
#35058=CARTESIAN_POINT('Ctrl Pts',(0.0983983261001443,-0.109911369421357,
3.5));
#35059=CARTESIAN_POINT('Ctrl Pts',(0.100785232866561,-0.107343907167555,
3.5));
#35060=CARTESIAN_POINT('Ctrl Pts',(0.103082837759472,-0.104696811464977,
3.5));
#35061=CARTESIAN_POINT('Ctrl Pts',(0.105281553373082,-0.101981102913922,
3.5));
#35062=CARTESIAN_POINT('Ctrl Pts',(0.111767020079616,-0.0939706820648148,
3.5));
#35063=CARTESIAN_POINT('Ctrl Pts',(0.117410242387804,-0.0853491014404185,
3.5));
#35064=CARTESIAN_POINT('Ctrl Pts',(0.122076804303227,-0.0762334533122014,
3.5));
#35065=CARTESIAN_POINT('Ctrl Pts',(0.124156859535273,-0.0721702796253988,
3.5));
#35066=CARTESIAN_POINT('Ctrl Pts',(0.126042226032514,-0.0680087185900064,
3.5));
#35067=CARTESIAN_POINT('Ctrl Pts',(0.127717516401833,-0.0637585923271345,
3.5));
#35068=CARTESIAN_POINT('Ctrl Pts',(0.128878955464437,-0.0608120806339354,
3.5));
#35069=CARTESIAN_POINT('Ctrl Pts',(0.129938690733468,-0.0578239271836136,
3.5));
#35070=CARTESIAN_POINT('Ctrl Pts',(0.130888204891735,-0.0548097446101512,
3.5));
#35071=CARTESIAN_POINT('Ctrl Pts',(0.132091470075251,-0.0509900428017762,
3.5));
#35072=CARTESIAN_POINT('Ctrl Pts',(0.133119907502104,-0.0471234083998808,
3.5));
#35073=CARTESIAN_POINT('Ctrl Pts',(0.13396498302397,-0.0432168875268929,
3.5));
#35074=CARTESIAN_POINT('Ctrl Pts',(0.135449870731708,-0.03635271423797,
3.5));
#35075=CARTESIAN_POINT('Ctrl Pts',(0.136369320260194,-0.0293652097985063,
3.5));
#35076=CARTESIAN_POINT('Ctrl Pts',(0.136739868479968,-0.022319296125407,
3.5));
#35077=CARTESIAN_POINT('Ctrl Pts',(0.136938614931574,-0.0185401649189451,
3.5));
#35078=CARTESIAN_POINT('Ctrl Pts',(0.13697923643291,-0.0147442545690828,
3.5));
#35079=CARTESIAN_POINT('Ctrl Pts',(0.136862895918197,-0.0109420689853019,
3.5));
#35080=CARTESIAN_POINT('Ctrl Pts',(0.136768618157157,-0.00786092786453014,
3.5));
#35081=CARTESIAN_POINT('Ctrl Pts',(0.136571008887471,-0.00477673741219634,
3.5));
#35082=CARTESIAN_POINT('Ctrl Pts',(0.136272480032331,-0.00170755776859209,
3.5));
#35083=CARTESIAN_POINT('Ctrl Pts',(0.135524862167375,0.00597871273026037,
3.5));
#35084=CARTESIAN_POINT('Ctrl Pts',(0.134145273604047,0.0135925891081728,
3.5));
#35085=CARTESIAN_POINT('Ctrl Pts',(0.132154756111308,0.0210469694652312,
3.5));
#35086=CARTESIAN_POINT('Ctrl Pts',(0.130956639638983,0.0255338508563019,
3.5));
#35087=CARTESIAN_POINT('Ctrl Pts',(0.129536820205507,0.0299628465144204,
3.5));
#35088=CARTESIAN_POINT('Ctrl Pts',(0.127896985354882,0.0343130630344241,
3.5));
#35089=CARTESIAN_POINT('Ctrl Pts',(0.126764260724531,0.0373179981946284,
3.5));
#35090=CARTESIAN_POINT('Ctrl Pts',(0.125525608395292,0.0402872565072415,
3.5));
#35091=CARTESIAN_POINT('Ctrl Pts',(0.124183958141022,0.0432071171955597,
3.5));
#35092=CARTESIAN_POINT('Ctrl Pts',(0.120305951421964,0.0516469019546402,
3.5));
#35093=CARTESIAN_POINT('Ctrl Pts',(0.115595095267004,0.0596252551381628,
3.5));
#35094=CARTESIAN_POINT('Ctrl Pts',(0.110076005567125,0.0669787038662309,
3.5));
#35095=CARTESIAN_POINT('Ctrl Pts',(0.106491490638639,0.0717545905024268,
3.5));
#35096=CARTESIAN_POINT('Ctrl Pts',(0.102565240148127,0.0762663779558996,
3.5));
#35097=CARTESIAN_POINT('Ctrl Pts',(0.0982968917172504,0.0804596491219306,
3.5));
#35098=CARTESIAN_POINT('Ctrl Pts',(0.0975400014439711,0.081203226224454,
3.5));
#35099=CARTESIAN_POINT('Ctrl Pts',(0.0967723418961243,0.0819367632413509,
3.5));
#35100=CARTESIAN_POINT('Ctrl Pts',(0.0959941578858439,0.0826601402795114,
3.5));
#35101=CARTESIAN_POINT('Origin',(0.,0.,4.11042117235887));
#35102=CARTESIAN_POINT('Ctrl Pts',(-0.154443265232512,0.000108744696557909,
3.98542117235887));
#35103=CARTESIAN_POINT('Ctrl Pts',(-0.154501375899708,0.00720215273278324,
3.98505427646906));
#35104=CARTESIAN_POINT('Ctrl Pts',(-0.150833043785448,0.0654047280234095,
3.98204082055362));
#35105=CARTESIAN_POINT('Ctrl Pts',(-0.0768181153328184,0.165435267997838,
3.97638080461255));
#35106=CARTESIAN_POINT('Ctrl Pts',(0.0973408978391562,0.154229954870798,
3.96844112453568));
#35107=CARTESIAN_POINT('Ctrl Pts',(0.182376570303567,0.00184388772387479,
3.9605014444588));
#35108=CARTESIAN_POINT('Ctrl Pts',(0.100432518024861,-0.152245093163996,
3.95256176438192));
#35109=CARTESIAN_POINT('Ctrl Pts',(-0.0734653243360244,-0.166934402953208,
3.94462208430505));
#35110=CARTESIAN_POINT('Ctrl Pts',(-0.150201443282177,-0.0675205906017345,
3.9389085536307));
#35111=CARTESIAN_POINT('Ctrl Pts',(-0.154485318877682,-0.00825665133948968,
3.93584158298197));
#35112=CARTESIAN_POINT('Ctrl Pts',(-0.154414683966261,-0.00012271194023455,
3.93542117235887));
#35113=CARTESIAN_POINT('Ctrl Pts',(-0.154145398954164,-0.000183190088064077,
3.98957882764113));
#35114=CARTESIAN_POINT('Ctrl Pts',(-0.153877225967651,0.0351591693674689,
3.9877594317095));
#35115=CARTESIAN_POINT('Ctrl Pts',(-0.124353035696744,0.122445639808398,
3.98329347575225));
#35116=CARTESIAN_POINT('Ctrl Pts',(0.0205691872966891,0.181176549232701,
3.97618095976937));
#35117=CARTESIAN_POINT('Ctrl Pts',(0.16339053139201,0.0810339956098913,
3.9682412796925));
#35118=CARTESIAN_POINT('Ctrl Pts',(0.156677599794682,-0.0933915431448235,
3.96030159961562));
#35119=CARTESIAN_POINT('Ctrl Pts',(0.00648228676056323,-0.182263829019595,
3.95236191953875));
#35120=CARTESIAN_POINT('Ctrl Pts',(-0.129338242603737,-0.114419911622588,
3.94545432888058));
#35121=CARTESIAN_POINT('Ctrl Pts',(-0.153936458995158,-0.0313143964796836,
3.94119329824804));
#35122=CARTESIAN_POINT('Ctrl Pts',(-0.154097159264761,8.62650376686723E-5,
3.93957882764113));
#35123=CARTESIAN_POINT('Ctrl Pts',(0.095811615272233,0.0825211298936557,
4.));
#35124=CARTESIAN_POINT('Ctrl Pts',(0.123256207240687,0.0506564342651108,
3.99735343997437));
#35125=CARTESIAN_POINT('Ctrl Pts',(0.143368215702842,-0.042067892211591,
3.99206031992312));
#35126=CARTESIAN_POINT('Ctrl Pts',(0.0422170408642446,-0.143478264550263,
3.98412063984626));
#35127=CARTESIAN_POINT('Ctrl Pts',(-0.0975844110283061,-0.113165467831369,
3.97618095976937));
#35128=CARTESIAN_POINT('Ctrl Pts',(-0.148038914743343,0.0205825766583269,
3.9682412796925));
#35129=CARTESIAN_POINT('Ctrl Pts',(-0.0629530180417037,0.135575435115532,
3.96030159961561));
#35130=CARTESIAN_POINT('Ctrl Pts',(0.0797715912622248,0.126392597494572,
3.95236191953875));
#35131=CARTESIAN_POINT('Ctrl Pts',(0.149458958618833,0.00151107973223563,
3.94442223946186));
#35132=CARTESIAN_POINT('Ctrl Pts',(0.0823051970462972,-0.124765988532646,
3.936482559385));
#35133=CARTESIAN_POINT('Ctrl Pts',(-0.0602053808314341,-0.136803987384531,
3.92854287930812));
#35134=CARTESIAN_POINT('Ctrl Pts',(-0.147593255628917,-0.0235905240738923,
3.92060319923124));
#35135=CARTESIAN_POINT('Ctrl Pts',(-0.0998481138804565,0.11122350451698,
3.91266351915437));
#35136=CARTESIAN_POINT('Ctrl Pts',(0.0393156975431816,0.144202992379161,
3.90472383907749));
#35137=CARTESIAN_POINT('Ctrl Pts',(0.142482946738445,0.0451539231751995,
3.89678415900061));
#35138=CARTESIAN_POINT('Ctrl Pts',(0.115196050889548,-0.0952372689088321,
3.88884447892374));
#35139=CARTESIAN_POINT('Ctrl Pts',(-0.0175617311292369,-0.148431271407445,
3.88090479884687));
#35140=CARTESIAN_POINT('Ctrl Pts',(-0.134240390927499,-0.0657250333201687,
3.87296511876998));
#35141=CARTESIAN_POINT('Ctrl Pts',(-0.128011600896121,0.0771575802637476,
3.86502543869311));
#35142=CARTESIAN_POINT('Ctrl Pts',(-0.00457829922889965,0.149396452528493,
3.85708575861623));
#35143=CARTESIAN_POINT('Ctrl Pts',(0.123046789066594,0.0848513369547663,
3.84914607853936));
#35144=CARTESIAN_POINT('Ctrl Pts',(0.138013034715666,-0.0573817376169498,
3.84120639846248));
#35145=CARTESIAN_POINT('Ctrl Pts',(0.0266176834030549,-0.147077395754537,
3.83326671838561));
#35146=CARTESIAN_POINT('Ctrl Pts',(-0.109148213688832,-0.102112335081275,
3.82532703830873));
#35147=CARTESIAN_POINT('Ctrl Pts',(-0.144980487747744,0.0363444586596486,
3.81738735823185));
#35148=CARTESIAN_POINT('Ctrl Pts',(-0.0480719232633252,0.141525092050256,
3.80944767815498));
#35149=CARTESIAN_POINT('Ctrl Pts',(0.0928502012748058,0.117128568782365,
3.8015079980781));
#35150=CARTESIAN_POINT('Ctrl Pts',(0.148760792417501,-0.0145082092888036,
3.79356831800123));
#35151=CARTESIAN_POINT('Ctrl Pts',(0.0684693840059589,-0.13286160073391,
3.78562863792435));
#35152=CARTESIAN_POINT('Ctrl Pts',(-0.0745110357927053,-0.129569931090983,
3.77768895784747));
#35153=CARTESIAN_POINT('Ctrl Pts',(-0.149270845181396,-0.00764697822290441,
3.7697492777706));
#35154=CARTESIAN_POINT('Ctrl Pts',(-0.0873616623012301,0.121277374051889,
3.76180959769372));
#35155=CARTESIAN_POINT('Ctrl Pts',(0.0545338724692569,0.139162919812538,
3.75386991761685));
#35156=CARTESIAN_POINT('Ctrl Pts',(0.146499433400264,0.0296340599732921,
3.74593023753997));
#35157=CARTESIAN_POINT('Ctrl Pts',(0.104333443683106,-0.107027071464762,
3.7379905574631));
#35158=CARTESIAN_POINT('Ctrl Pts',(-0.0333578751151315,-0.14569664946404,
3.73005087738622));
#35159=CARTESIAN_POINT('Ctrl Pts',(-0.14050748182764,-0.0509696875349592,
3.72211119730934));
#35160=CARTESIAN_POINT('Ctrl Pts',(-0.119011632529845,0.0904239615350441,
3.71417151723247));
#35161=CARTESIAN_POINT('Ctrl Pts',(0.0114485618600744,0.149027487159785,
3.70623183715559));
#35162=CARTESIAN_POINT('Ctrl Pts',(0.131426713281372,0.0711848335798314,
3.69829215707872));
#35163=CARTESIAN_POINT('Ctrl Pts',(0.131073553936911,-0.0718330352678932,
3.69035247700184));
#35164=CARTESIAN_POINT('Ctrl Pts',(0.0107124284623447,-0.149082210133256,
3.68241279692496));
#35165=CARTESIAN_POINT('Ctrl Pts',(-0.119456752931603,-0.0898351026331364,
3.67447311684809));
#35166=CARTESIAN_POINT('Ctrl Pts',(-0.140254047194737,0.0516629823793918,
3.66653343677121));
#35167=CARTESIAN_POINT('Ctrl Pts',(-0.0326379242804108,0.145859615472823,
3.65859375669434));
#35168=CARTESIAN_POINT('Ctrl Pts',(0.10486073980172,0.10651050023316,3.65065407661746));
#35169=CARTESIAN_POINT('Ctrl Pts',(0.146351295051501,-0.0303572067245441,
3.64271439654059));
#35170=CARTESIAN_POINT('Ctrl Pts',(0.0538459306115186,-0.139430547008859,
3.63477471646371));
#35171=CARTESIAN_POINT('Ctrl Pts',(-0.0879595415059408,-0.12084444509365,
3.62683503638684));
#35172=CARTESIAN_POINT('Ctrl Pts',(-0.149231261493045,0.00838407713103302,
3.61889535630996));
#35173=CARTESIAN_POINT('Ctrl Pts',(-0.0738702226095378,0.12993634123263,
3.61095567623308));
#35174=CARTESIAN_POINT('Ctrl Pts',(0.0691246960538845,0.132521821325185,
3.60301599615621));
#35175=CARTESIAN_POINT('Ctrl Pts',(0.148830647021129,0.0137733814668988,
3.59507631607933));
#35176=CARTESIAN_POINT('Ctrl Pts',(0.0922705776859184,-0.11758574481156,
3.58713663600245));
#35177=CARTESIAN_POINT('Ctrl Pts',(-0.0487702109612334,-0.141285857774966,
3.57919695592558));
#35178=CARTESIAN_POINT('Ctrl Pts',(-0.145158345123895,-0.0356282001147357,
3.5712572758487));
#35179=CARTESIAN_POINT('Ctrl Pts',(-0.108642326262961,0.10265050841275,
3.56331759577183));
#35180=CARTESIAN_POINT('Ctrl Pts',(0.0273432144577738,0.14694341587319,
3.55537791569495));
#35181=CARTESIAN_POINT('Ctrl Pts',(0.138295730077318,0.0567008676982971,
3.54743823561807));
#35182=CARTESIAN_POINT('Ctrl Pts',(0.122624304118183,-0.0854607729482632,
3.5394985555412));
#35183=CARTESIAN_POINT('Ctrl Pts',(-0.00531228376040394,-0.149366579646122,
3.53155887546432));
#35184=CARTESIAN_POINT('Ctrl Pts',(-0.128398465432132,-0.0765350583850204,
3.52361919538745));
#35185=CARTESIAN_POINT('Ctrl Pts',(-0.133899765542225,0.0664079477775043,
3.51567951531057));
#35186=CARTESIAN_POINT('Ctrl Pts',(-0.0168566046022346,0.148475571278638,
3.5077398352337));
#35187=CARTESIAN_POINT('Ctrl Pts',(0.115720245650148,0.0947476421044766,
3.49980015515682));
#35188=CARTESIAN_POINT('Ctrl Pts',(0.142146925240749,-0.0460261281615502,
3.49186047507995));
#35189=CARTESIAN_POINT('Ctrl Pts',(0.0732860006472317,-0.111298378536925,
3.48656735502869));
#35190=CARTESIAN_POINT('Ctrl Pts',(0.0326585063531174,-0.122159831625553,
3.48392079500307));
#35191=CARTESIAN_POINT('Ctrl Pts',(0.102845629995659,0.0885794229410745,
4.00535973499898));
#35192=CARTESIAN_POINT('Ctrl Pts',(0.132305068112318,0.0543753790239966,
4.00271317497335));
#35193=CARTESIAN_POINT('Ctrl Pts',(0.153893600722808,-0.0451563087084747,
3.9974200549221));
#35194=CARTESIAN_POINT('Ctrl Pts',(0.0453164071172279,-0.154011728812092,
3.98948037484522));
#35195=CARTESIAN_POINT('Ctrl Pts',(-0.104748575644461,-0.121473516543913,
3.98154069476835));
#35196=CARTESIAN_POINT('Ctrl Pts',(-0.158907199376537,0.0220936475952833,
3.97360101469147));
#35197=CARTESIAN_POINT('Ctrl Pts',(-0.067574717138742,0.145528712742967,
3.9656613346146));
#35198=CARTESIAN_POINT('Ctrl Pts',(0.0856280267878686,0.135671716619981,
3.95772165453772));
#35199=CARTESIAN_POINT('Ctrl Pts',(0.160431495847078,0.00162201572944855,
3.94978197446085));
#35200=CARTESIAN_POINT('Ctrl Pts',(0.0883476373724852,-0.133925690076429,
3.94184229438397));
#35201=CARTESIAN_POINT('Ctrl Pts',(-0.0646253619996309,-0.146847459240757,
3.93390261430709));
#35202=CARTESIAN_POINT('Ctrl Pts',(-0.158428822175023,-0.0253224236269645,
3.92596293423022));
#35203=CARTESIAN_POINT('Ctrl Pts',(-0.107178468359357,0.119388983891694,
3.91802325415334));
#35204=CARTESIAN_POINT('Ctrl Pts',(0.0422020615251973,0.15478966257228,
3.91008357407647));
#35205=CARTESIAN_POINT('Ctrl Pts',(0.152943339691301,0.0484689007959436,
3.90214389399959));
#35206=CARTESIAN_POINT('Ctrl Pts',(0.123653174963026,-0.102229117964087,
3.89420421392272));
#35207=CARTESIAN_POINT('Ctrl Pts',(-0.0188510265344017,-0.159328360925561,
3.88626453384584));
#35208=CARTESIAN_POINT('Ctrl Pts',(-0.144095656216364,-0.0705502400631941,
3.87832485376896));
#35209=CARTESIAN_POINT('Ctrl Pts',(-0.137409579240545,0.0828221080358456,
3.87038517369209));
#35210=CARTESIAN_POINT('Ctrl Pts',(-0.00491441530514796,0.160364400868861,
3.86244549361521));
#35211=CARTESIAN_POINT('Ctrl Pts',(0.13208027549207,0.0910807022748934,
3.85450581353834));
#35212=CARTESIAN_POINT('Ctrl Pts',(0.148145268844653,-0.0615944208715485,
3.84656613346146));
#35213=CARTESIAN_POINT('Ctrl Pts',(0.0285718220158795,-0.157875090421108,
3.83862645338458));
#35214=CARTESIAN_POINT('Ctrl Pts',(-0.117161335479353,-0.109608917477515,
3.83068677330771));
#35215=CARTESIAN_POINT('Ctrl Pts',(-0.155624237803826,0.0390126889843388,
3.82274709323083));
#35216=CARTESIAN_POINT('Ctrl Pts',(-0.0516011260124583,0.151915164051309,
3.81480741315396));
#35217=CARTESIAN_POINT('Ctrl Pts',(0.0996668036354316,0.125727568757556,
3.80686773307708));
#35218=CARTESIAN_POINT('Ctrl Pts',(0.159682073737726,-0.0155733302290782,
3.7989280530002));
#35219=CARTESIAN_POINT('Ctrl Pts',(0.0734960673974602,-0.142615642068929,
3.79098837292333));
#35220=CARTESIAN_POINT('Ctrl Pts',(-0.0799812673646754,-0.139082314327793,
3.78304869284645));
#35221=CARTESIAN_POINT('Ctrl Pts',(-0.160229572051837,-0.00820838152726148,
3.77510901276958));
#35222=CARTESIAN_POINT('Ctrl Pts',(-0.0937753232873622,0.13018095878194,
3.7671693326927));
#35223=CARTESIAN_POINT('Ctrl Pts',(0.0585374795557702,0.149379572815778,
3.75922965261583));
#35224=CARTESIAN_POINT('Ctrl Pts',(0.157254696930506,0.0318096460290618,
3.75128997253895));
#35225=CARTESIAN_POINT('Ctrl Pts',(0.111993088882986,-0.11488446948847,
3.74335029246207));
#35226=CARTESIAN_POINT('Ctrl Pts',(-0.0358068452534112,-0.156392976569809,
3.7354106123852));
#35227=CARTESIAN_POINT('Ctrl Pts',(-0.15082284592122,-0.0547116297989597,
3.72747093230832));
#35228=CARTESIAN_POINT('Ctrl Pts',(-0.127748877728095,0.0970624413788584,
3.71953125223145));
#35229=CARTESIAN_POINT('Ctrl Pts',(0.0122890586250752,0.1599683478884,3.71159157215457));
#35230=CARTESIAN_POINT('Ctrl Pts',(0.141075412279359,0.0764108718431722,
3.7036518920777));
#35231=CARTESIAN_POINT('Ctrl Pts',(0.140696325723237,-0.0771066612919101,
3.69571221200082));
#35232=CARTESIAN_POINT('Ctrl Pts',(0.0114988819556263,-0.160027088351817,
3.68777253192394));
#35233=CARTESIAN_POINT('Ctrl Pts',(-0.128226676667323,-0.0964303513700096,
3.67983285184707));
#35234=CARTESIAN_POINT('Ctrl Pts',(-0.150550805371548,0.0554558229204912,
3.67189317177019));
#35235=CARTESIAN_POINT('Ctrl Pts',(-0.035034039190677,0.156567906736611,
3.66395349169332));
#35236=CARTESIAN_POINT('Ctrl Pts',(0.112559096473601,0.114329974153006,
3.65601381161644));
#35237=CARTESIAN_POINT('Ctrl Pts',(0.157095682997156,-0.0325858826367059,
3.64807413153956));
#35238=CARTESIAN_POINT('Ctrl Pts',(0.0577990324107298,-0.14966684787665,
3.64013445146269));
#35239=CARTESIAN_POINT('Ctrl Pts',(-0.0944170958250141,-0.129716246321693,
3.63219477138581));
#35240=CARTESIAN_POINT('Ctrl Pts',(-0.160187082324945,0.00899959459010582,
3.62425509130894));
#35241=CARTESIAN_POINT('Ctrl Pts',(-0.0792934088483033,0.139475624489065,
3.61631541123206));
#35242=CARTESIAN_POINT('Ctrl Pts',(0.0741994892135014,0.142250917737222,
3.60837573115519));
#35243=CARTESIAN_POINT('Ctrl Pts',(0.159757056720716,0.0147845549843712,
3.60043605107831));
#35244=CARTESIAN_POINT('Ctrl Pts',(0.099044626950589,-0.126218308388737,
3.59249637100143));
#35245=CARTESIAN_POINT('Ctrl Pts',(-0.0523506785380631,-0.151658366379244,
3.58455669092456));
#35246=CARTESIAN_POINT('Ctrl Pts',(-0.155815152588506,-0.0382438462810607,
3.57661701084768));
#35247=CARTESIAN_POINT('Ctrl Pts',(-0.116618308301774,0.110186600832138,
3.5686773307708));
#35248=CARTESIAN_POINT('Ctrl Pts',(0.0293506179707539,0.157731274399797,
3.56073765069393));
#35249=CARTESIAN_POINT('Ctrl Pts',(0.148448718300998,0.06086356485237,3.55279797061705));
#35250=CARTESIAN_POINT('Ctrl Pts',(0.131626773789177,-0.0917348800435817,
3.54485829054018));
#35251=CARTESIAN_POINT('Ctrl Pts',(-0.00570228534924597,-0.160332334867275,
3.5369186104633));
#35252=CARTESIAN_POINT('Ctrl Pts',(-0.137824845456608,-0.0821538836809814,
3.52897893038643));
#35253=CARTESIAN_POINT('Ctrl Pts',(-0.143730023800696,0.0712832907209694,
3.52103925030955));
#35254=CARTESIAN_POINT('Ctrl Pts',(-0.0180941331067087,0.159375913074104,
3.51309957023267));
#35255=CARTESIAN_POINT('Ctrl Pts',(0.124215853509266,0.101703545182399,
3.5051598901558));
#35256=CARTESIAN_POINT('Ctrl Pts',(0.152582649157857,-0.0494051387567767,
3.49722021007893));
#35257=CARTESIAN_POINT('Ctrl Pts',(0.0786662962002181,-0.119469354791712,
3.49192709002767));
#35258=CARTESIAN_POINT('Ctrl Pts',(0.0350561322973228,-0.131128202024318,
3.48928053000205));
#35259=CARTESIAN_POINT('Ctrl Pts',(0.109879644719085,0.0946377159884933,
4.01071946999795));
#35260=CARTESIAN_POINT('Ctrl Pts',(0.141353928983949,0.0580943237828825,
4.00807290997233));
#35261=CARTESIAN_POINT('Ctrl Pts',(0.164418985742774,-0.0482447252053583,
4.00277978992107));
#35262=CARTESIAN_POINT('Ctrl Pts',(0.0484157733702112,-0.164545193073921,
3.99484010984421));
#35263=CARTESIAN_POINT('Ctrl Pts',(-0.111912740260616,-0.129781565256457,
3.98690042976732));
#35264=CARTESIAN_POINT('Ctrl Pts',(-0.16977548400973,0.0236047185322397,
3.97896074969046));
#35265=CARTESIAN_POINT('Ctrl Pts',(-0.0721964162357802,0.155481990370402,
3.97102106961357));
#35266=CARTESIAN_POINT('Ctrl Pts',(0.0914844623135124,0.14495083574539,
3.9630813895367));
#35267=CARTESIAN_POINT('Ctrl Pts',(0.171404033075322,0.0017329517266617,
3.95514170945982));
#35268=CARTESIAN_POINT('Ctrl Pts',(0.0943900776986731,-0.143085391620212,
3.94720202938295));
#35269=CARTESIAN_POINT('Ctrl Pts',(-0.0690453431678277,-0.156890931096983,
3.93926234930607));
#35270=CARTESIAN_POINT('Ctrl Pts',(-0.169264388721129,-0.0270543231800365,
3.9313226692292));
#35271=CARTESIAN_POINT('Ctrl Pts',(-0.114508822838256,0.127554463266409,
3.92338298915232));
#35272=CARTESIAN_POINT('Ctrl Pts',(0.0450884255072127,0.165376332765398,
3.91544330907545));
#35273=CARTESIAN_POINT('Ctrl Pts',(0.163403732644156,0.0517838784166879,
3.90750362899857));
#35274=CARTESIAN_POINT('Ctrl Pts',(0.132110299036504,-0.109220967019342,
3.89956394892169));
#35275=CARTESIAN_POINT('Ctrl Pts',(-0.0201403219395664,-0.170225450443677,
3.89162426884482));
#35276=CARTESIAN_POINT('Ctrl Pts',(-0.153950921505229,-0.0753754468062197,
3.88368458876794));
#35277=CARTESIAN_POINT('Ctrl Pts',(-0.146807557584968,0.0884866358079437,
3.87574490869107));
#35278=CARTESIAN_POINT('Ctrl Pts',(-0.00525053138139654,0.171332349209229,
3.86780522861419));
#35279=CARTESIAN_POINT('Ctrl Pts',(0.141113761917547,0.0973100675950205,
3.85986554853731));
#35280=CARTESIAN_POINT('Ctrl Pts',(0.15827750297364,-0.0658071041261473,
3.85192586846044));
#35281=CARTESIAN_POINT('Ctrl Pts',(0.0305259606287044,-0.16867278508768,
3.84398618838356));
#35282=CARTESIAN_POINT('Ctrl Pts',(-0.125174457269873,-0.117105499873754,
3.83604650830669));
#35283=CARTESIAN_POINT('Ctrl Pts',(-0.166267987859908,0.0416809193090289,
3.82810682822981));
#35284=CARTESIAN_POINT('Ctrl Pts',(-0.0551303287615912,0.162305236052362,
3.82016714815293));
#35285=CARTESIAN_POINT('Ctrl Pts',(0.106483405996057,0.134326568732747,
3.81222746807606));
#35286=CARTESIAN_POINT('Ctrl Pts',(0.170603355057952,-0.0166384511693528,
3.80428778799918));
#35287=CARTESIAN_POINT('Ctrl Pts',(0.0785227507889612,-0.152369683403947,
3.79634810792231));
#35288=CARTESIAN_POINT('Ctrl Pts',(-0.0854514989366454,-0.148594697564603,
3.78840842784543));
#35289=CARTESIAN_POINT('Ctrl Pts',(-0.171188298922279,-0.00876978483161878,
3.78046874776855));
#35290=CARTESIAN_POINT('Ctrl Pts',(-0.100188984273494,0.139084543511992,
3.77252906769168));
#35291=CARTESIAN_POINT('Ctrl Pts',(0.0625410866422834,0.159596225819019,
3.7645893876148));
#35292=CARTESIAN_POINT('Ctrl Pts',(0.168009960460748,0.0339852320848313,
3.75664970753793));
#35293=CARTESIAN_POINT('Ctrl Pts',(0.119652734082865,-0.122741867512178,
3.74871002746105));
#35294=CARTESIAN_POINT('Ctrl Pts',(-0.0382558153916907,-0.167089303675579,
3.74077034738417));
#35295=CARTESIAN_POINT('Ctrl Pts',(-0.161138210014801,-0.0584535720629604,
3.7328306673073));
#35296=CARTESIAN_POINT('Ctrl Pts',(-0.136486122926345,0.103700921222673,
3.72489098723042));
#35297=CARTESIAN_POINT('Ctrl Pts',(0.0131295553900761,0.170909208617015,
3.71695130715355));
#35298=CARTESIAN_POINT('Ctrl Pts',(0.150724111277345,0.081636910106513,
3.70901162707667));
#35299=CARTESIAN_POINT('Ctrl Pts',(0.150319097509564,-0.0823802873159272,
3.7010719469998));
#35300=CARTESIAN_POINT('Ctrl Pts',(0.0122853354489075,-0.170971966570378,
3.69313226692292));
#35301=CARTESIAN_POINT('Ctrl Pts',(-0.136996600403042,-0.103025600106883,
3.68519258684605));
#35302=CARTESIAN_POINT('Ctrl Pts',(-0.16084756354836,0.0592486634615907,
3.67725290676916));
#35303=CARTESIAN_POINT('Ctrl Pts',(-0.037430154100943,0.1672761980004,3.66931322669229));
#35304=CARTESIAN_POINT('Ctrl Pts',(0.120257453145481,0.122149448072851,
3.66137354661541));
#35305=CARTESIAN_POINT('Ctrl Pts',(0.167840070942811,-0.0348145585488677,
3.65343386653854));
#35306=CARTESIAN_POINT('Ctrl Pts',(0.0617521342099411,-0.159903148744442,
3.64549418646166));
#35307=CARTESIAN_POINT('Ctrl Pts',(-0.100874650144087,-0.138588047549736,
3.63755450638479));
#35308=CARTESIAN_POINT('Ctrl Pts',(-0.171142903156845,0.00961511204917869,
3.62961482630791));
#35309=CARTESIAN_POINT('Ctrl Pts',(-0.0847165950870686,0.149014907745501,
3.62167514623104));
#35310=CARTESIAN_POINT('Ctrl Pts',(0.0792742823731183,0.15198001414926,
3.61373546615416));
#35311=CARTESIAN_POINT('Ctrl Pts',(0.170683466420304,0.0157957285018435,
3.60579578607728));
#35312=CARTESIAN_POINT('Ctrl Pts',(0.10581867621526,-0.134850871965913,
3.59785610600041));
#35313=CARTESIAN_POINT('Ctrl Pts',(-0.0559311461148929,-0.162030874983522,
3.58991642592353));
#35314=CARTESIAN_POINT('Ctrl Pts',(-0.166471960053118,-0.0408594924473857,
3.58197674584666));
#35315=CARTESIAN_POINT('Ctrl Pts',(-0.124594290340586,0.117722693251527,
3.57403706576978));
#35316=CARTESIAN_POINT('Ctrl Pts',(0.0313580214837342,0.168519132926404,
3.56609738569291));
#35317=CARTESIAN_POINT('Ctrl Pts',(0.158601706524679,0.065026262006443,
3.55815770561603));
#35318=CARTESIAN_POINT('Ctrl Pts',(0.14062924346017,-0.0980089871389004,
3.55021802553916));
#35319=CARTESIAN_POINT('Ctrl Pts',(-0.00609228693808808,-0.171298090088428,
3.54227834546228));
#35320=CARTESIAN_POINT('Ctrl Pts',(-0.147251225481083,-0.0877727089769424,
3.5343386653854));
#35321=CARTESIAN_POINT('Ctrl Pts',(-0.153560282059167,0.0761586336644345,
3.52639898530853));
#35322=CARTESIAN_POINT('Ctrl Pts',(-0.0193316616111828,0.17027625486957,
3.51845930523165));
#35323=CARTESIAN_POINT('Ctrl Pts',(0.132711461368385,0.10865944826032,3.51051962515478));
#35324=CARTESIAN_POINT('Ctrl Pts',(0.163018373074965,-0.0527841493520032,
3.5025799450779));
#35325=CARTESIAN_POINT('Ctrl Pts',(0.0840465917532045,-0.127640331046499,
3.49728682502665));
#35326=CARTESIAN_POINT('Ctrl Pts',(0.0374537582415282,-0.140096572423083,
3.49464026500102));
#35327=CARTESIAN_POINT('Ctrl Pts',(0.116913659442511,0.100696009035912,
4.01607920499693));
#35328=CARTESIAN_POINT('Ctrl Pts',(0.15040278985558,0.0618132685417683,
4.01343264497131));
#35329=CARTESIAN_POINT('Ctrl Pts',(0.17494437076274,-0.0513331417022419,
4.00813952492005));
#35330=CARTESIAN_POINT('Ctrl Pts',(0.0515151396231945,-0.17507865733575,
4.00019984484318));
#35331=CARTESIAN_POINT('Ctrl Pts',(-0.119076904876771,-0.138089613969001,
3.9922601647663));
#35332=CARTESIAN_POINT('Ctrl Pts',(-0.180643768642924,0.0251157894691961,
3.98432048468943));
#35333=CARTESIAN_POINT('Ctrl Pts',(-0.0768181153328184,0.165435267997838,
3.97638080461255));
#35334=CARTESIAN_POINT('Ctrl Pts',(0.0973408978391562,0.154229954870798,
3.96844112453568));
#35335=CARTESIAN_POINT('Ctrl Pts',(0.182376570303567,0.00184388772387479,
3.9605014444588));
#35336=CARTESIAN_POINT('Ctrl Pts',(0.100432518024861,-0.152245093163996,
3.95256176438192));
#35337=CARTESIAN_POINT('Ctrl Pts',(-0.0734653243360244,-0.166934402953208,
3.94462208430505));
#35338=CARTESIAN_POINT('Ctrl Pts',(-0.180099955267235,-0.0287862227331087,
3.93668240422817));
#35339=CARTESIAN_POINT('Ctrl Pts',(-0.121839177317157,0.135719942641123,
3.9287427241513));
#35340=CARTESIAN_POINT('Ctrl Pts',(0.0479747894892283,0.175963002958517,
3.92080304407442));
#35341=CARTESIAN_POINT('Ctrl Pts',(0.173864125597012,0.0550988560374321,
3.91286336399754));
#35342=CARTESIAN_POINT('Ctrl Pts',(0.140567423109983,-0.116212816074597,
3.90492368392067));
#35343=CARTESIAN_POINT('Ctrl Pts',(-0.0214296173447312,-0.181122539961793,
3.89698400384379));
#35344=CARTESIAN_POINT('Ctrl Pts',(-0.163806186794094,-0.0802006535492451,
3.88904432376692));
#35345=CARTESIAN_POINT('Ctrl Pts',(-0.156205535929391,0.0941511635800416,
3.88110464369004));
#35346=CARTESIAN_POINT('Ctrl Pts',(-0.005586647457645,0.182300297549597,
3.87316496361317));
#35347=CARTESIAN_POINT('Ctrl Pts',(0.150147248343024,0.103539432915148,
3.86522528353629));
#35348=CARTESIAN_POINT('Ctrl Pts',(0.168409737102627,-0.0700197873807462,
3.85728560345941));
#35349=CARTESIAN_POINT('Ctrl Pts',(0.0324800992415292,-0.179470479754251,
3.84934592338254));
#35350=CARTESIAN_POINT('Ctrl Pts',(-0.133187579060394,-0.124602082269994,
3.84140624330566));
#35351=CARTESIAN_POINT('Ctrl Pts',(-0.17691173791599,0.0443491496337192,
3.83346656322879));
#35352=CARTESIAN_POINT('Ctrl Pts',(-0.0586595315107243,0.172695308053416,
3.82552688315191));
#35353=CARTESIAN_POINT('Ctrl Pts',(0.113300008356683,0.142925568707939,
3.81758720307504));
#35354=CARTESIAN_POINT('Ctrl Pts',(0.181524636378177,-0.0177035721096275,
3.80964752299816));
#35355=CARTESIAN_POINT('Ctrl Pts',(0.0835494341804624,-0.162123724738966,
3.80170784292129));
#35356=CARTESIAN_POINT('Ctrl Pts',(-0.0909217305086156,-0.158107080801413,
3.7937681628444));
#35357=CARTESIAN_POINT('Ctrl Pts',(-0.18214702579272,-0.00933118813597588,
3.78582848276753));
#35358=CARTESIAN_POINT('Ctrl Pts',(-0.106602645259627,0.147988128242044,
3.77788880269065));
#35359=CARTESIAN_POINT('Ctrl Pts',(0.0665446937287967,0.169812878822259,
3.76994912261378));
#35360=CARTESIAN_POINT('Ctrl Pts',(0.178765223990991,0.0361608181406009,
3.7620094425369));
#35361=CARTESIAN_POINT('Ctrl Pts',(0.127312379282745,-0.130599265535886,
3.75406976246003));
#35362=CARTESIAN_POINT('Ctrl Pts',(-0.0407047855299705,-0.177785630781348,
3.74613008238315));
#35363=CARTESIAN_POINT('Ctrl Pts',(-0.171453574108382,-0.0621955143269609,
3.73819040230628));
#35364=CARTESIAN_POINT('Ctrl Pts',(-0.145223368124595,0.110339401066487,
3.7302507222294));
#35365=CARTESIAN_POINT('Ctrl Pts',(0.0139700521550768,0.18185006934563,
3.72231104215253));
#35366=CARTESIAN_POINT('Ctrl Pts',(0.160372810275332,0.0868629483698537,
3.71437136207565));
#35367=CARTESIAN_POINT('Ctrl Pts',(0.15994186929589,-0.087653913339944,
3.70643168199877));
#35368=CARTESIAN_POINT('Ctrl Pts',(0.013071788942189,-0.181916844788939,
3.6984920019219));
#35369=CARTESIAN_POINT('Ctrl Pts',(-0.145766524138762,-0.109620848843756,
3.69055232184502));
#35370=CARTESIAN_POINT('Ctrl Pts',(-0.171144321725171,0.06304150400269,
3.68261264176815));
#35371=CARTESIAN_POINT('Ctrl Pts',(-0.039826269011209,0.177984489264188,
3.67467296169127));
#35372=CARTESIAN_POINT('Ctrl Pts',(0.127955809817362,0.129968921992697,
3.66673328161439));
#35373=CARTESIAN_POINT('Ctrl Pts',(0.178584458888466,-0.0370432344610292,
3.65879360153752));
#35374=CARTESIAN_POINT('Ctrl Pts',(0.0657052360091523,-0.170139449612234,
3.65085392146064));
#35375=CARTESIAN_POINT('Ctrl Pts',(-0.107332204463161,-0.147459848777779,
3.64291424138377));
#35376=CARTESIAN_POINT('Ctrl Pts',(-0.182098723988745,0.0102306295082514,
3.63497456130689));
#35377=CARTESIAN_POINT('Ctrl Pts',(-0.0901397813258339,0.158554191001936,
3.62703488123002));
#35378=CARTESIAN_POINT('Ctrl Pts',(0.0843490755327352,0.161709110561297,
3.61909520115314));
#35379=CARTESIAN_POINT('Ctrl Pts',(0.181609876119891,0.0168069020193158,
3.61115552107626));
#35380=CARTESIAN_POINT('Ctrl Pts',(0.11259272547993,-0.14348343554309,3.60321584099938));
#35381=CARTESIAN_POINT('Ctrl Pts',(-0.0595116136917225,-0.1724033835878,
3.59527616092251));
#35382=CARTESIAN_POINT('Ctrl Pts',(-0.17712876751773,-0.0434751386137106,
3.58733648084563));
#35383=CARTESIAN_POINT('Ctrl Pts',(-0.132570272379398,0.125258785670915,
3.57939680076876));
#35384=CARTESIAN_POINT('Ctrl Pts',(0.0333654249967142,0.179306991453011,
3.57145712069188));
#35385=CARTESIAN_POINT('Ctrl Pts',(0.16875469474836,0.0691889591605158,
3.56351744061501));
#35386=CARTESIAN_POINT('Ctrl Pts',(0.149631713131164,-0.104283094234219,
3.55557776053813));
#35387=CARTESIAN_POINT('Ctrl Pts',(-0.00648228852693025,-0.182263845309582,
3.54763808046125));
#35388=CARTESIAN_POINT('Ctrl Pts',(-0.156677605505559,-0.0933915342729034,
3.53969840038438));
#35389=CARTESIAN_POINT('Ctrl Pts',(-0.163390540317638,0.0810339766078996,
3.5317587203075));
#35390=CARTESIAN_POINT('Ctrl Pts',(-0.0205691901156568,0.181176596665036,
3.52381904023063));
#35391=CARTESIAN_POINT('Ctrl Pts',(0.141207069227503,0.115615351338242,
3.51587936015375));
#35392=CARTESIAN_POINT('Ctrl Pts',(0.173454096992073,-0.0561631599472297,
3.50793968007688));
#35393=CARTESIAN_POINT('Ctrl Pts',(0.089426887306191,-0.135811307301286,
3.50264656002563));
#35394=CARTESIAN_POINT('Ctrl Pts',(0.0398513841857336,-0.149064942821849,
3.5));
#35395=CARTESIAN_POINT('Ctrl Pts',(0.095811615272233,0.0825211298936557,
4.));
#35396=CARTESIAN_POINT('Ctrl Pts',(0.102493030557671,0.0762815759767258,
4.));
#35397=CARTESIAN_POINT('Ctrl Pts',(0.10839405706188,0.0693097484661253,
4.));
#35398=CARTESIAN_POINT('Ctrl Pts',(0.11350885289652,0.0617853075148104,
4.));
#35399=CARTESIAN_POINT('Ctrl Pts',(0.117424080053794,0.0560255672420171,
4.));
#35400=CARTESIAN_POINT('Ctrl Pts',(0.120878299816185,0.0499406938168944,
4.));
#35401=CARTESIAN_POINT('Ctrl Pts',(0.123857056765335,0.0435961076613069,
4.));
#35402=CARTESIAN_POINT('Ctrl Pts',(0.125170781948423,0.0407979462969676,
4.));
#35403=CARTESIAN_POINT('Ctrl Pts',(0.126390002992329,0.0379525898756446,
4.));
#35404=CARTESIAN_POINT('Ctrl Pts',(0.12751038950843,0.0350750832122783,
4.));
#35405=CARTESIAN_POINT('Ctrl Pts',(0.131085166597008,0.0258939258664803,
4.));
#35406=CARTESIAN_POINT('Ctrl Pts',(0.133669431833427,0.0163619242015854,
4.));
#35407=CARTESIAN_POINT('Ctrl Pts',(0.135230958047781,0.0066616777752228,
4.));
#35408=CARTESIAN_POINT('Ctrl Pts',(0.135923073683569,0.00236223524203686,
4.));
#35409=CARTESIAN_POINT('Ctrl Pts',(0.136413711726375,-0.0019706858607116,
4.));
#35410=CARTESIAN_POINT('Ctrl Pts',(0.136697089502038,-0.00632254181082518,
4.));
#35411=CARTESIAN_POINT('Ctrl Pts',(0.136879678085431,-0.00912656979504798,
4.));
#35412=CARTESIAN_POINT('Ctrl Pts',(0.136975856810266,-0.011936494905405,
4.));
#35413=CARTESIAN_POINT('Ctrl Pts',(0.136984537674321,-0.0147391030393356,
4.));
#35414=CARTESIAN_POINT('Ctrl Pts',(0.137010531466213,-0.0231311723225325,
4.));
#35415=CARTESIAN_POINT('Ctrl Pts',(0.136255503035819,-0.0314800211532621,
4.));
#35416=CARTESIAN_POINT('Ctrl Pts',(0.134693290097439,-0.0396806821547801,
4.));
#35417=CARTESIAN_POINT('Ctrl Pts',(0.133704762250079,-0.0448698478361003,
4.));
#35418=CARTESIAN_POINT('Ctrl Pts',(0.132392592878428,-0.0499999054788172,
4.));
#35419=CARTESIAN_POINT('Ctrl Pts',(0.130776991260223,-0.0550529928649125,
4.));
#35420=CARTESIAN_POINT('Ctrl Pts',(0.129445892801333,-0.0592162449664668,
4.));
#35421=CARTESIAN_POINT('Ctrl Pts',(0.127906314848104,-0.0633316423760335,
4.));
#35422=CARTESIAN_POINT('Ctrl Pts',(0.126180878863323,-0.0673610722009708,
4.));
#35423=CARTESIAN_POINT('Ctrl Pts',(0.122312843187174,-0.0763941388895448,
4.));
#35424=CARTESIAN_POINT('Ctrl Pts',(0.117508253438465,-0.0850205194401279,
4.));
#35425=CARTESIAN_POINT('Ctrl Pts',(0.111900166266883,-0.0931314900308112,
4.));
#35426=CARTESIAN_POINT('Ctrl Pts',(0.108605841530307,-0.097896068439994,
4.));
#35427=CARTESIAN_POINT('Ctrl Pts',(0.105033346987346,-0.102482765945667,
4.));
#35428=CARTESIAN_POINT('Ctrl Pts',(0.101203104491781,-0.106867390005116,
4.));
#35429=CARTESIAN_POINT('Ctrl Pts',(0.0988795404734533,-0.109527261987172,
4.));
#35430=CARTESIAN_POINT('Ctrl Pts',(0.0964620699804362,-0.112111128650417,
4.));
#35431=CARTESIAN_POINT('Ctrl Pts',(0.0939639375491823,-0.114605366763082,
4.));
#35432=CARTESIAN_POINT('Ctrl Pts',(0.0874788757256353,-0.121080319075824,
4.));
#35433=CARTESIAN_POINT('Ctrl Pts',(0.0804377540716352,-0.126968968726175,
4.));
#35434=CARTESIAN_POINT('Ctrl Pts',(0.0729230547225638,-0.132178932127324,
4.));
#35435=CARTESIAN_POINT('Ctrl Pts',(0.0694491809116136,-0.134587379168854,
4.));
#35436=CARTESIAN_POINT('Ctrl Pts',(0.0658808132415588,-0.136845565695848,
4.));
#35437=CARTESIAN_POINT('Ctrl Pts',(0.0622290543017492,-0.138943290379685,
4.));
#35438=CARTESIAN_POINT('Ctrl Pts',(0.0562216582547972,-0.142394192583524,
4.));
#35439=CARTESIAN_POINT('Ctrl Pts',(0.0499865922958981,-0.145412833318798,
4.));
#35440=CARTESIAN_POINT('Ctrl Pts',(0.0435567401413007,-0.147956905966761,
4.));
#35441=CARTESIAN_POINT('Ctrl Pts',(0.0423577886630555,-0.148431290072134,
4.));
#35442=CARTESIAN_POINT('Ctrl Pts',(0.0411520494229064,-0.148889152887265,
4.));
#35443=CARTESIAN_POINT('Ctrl Pts',(0.0399398308045252,-0.149330586455588,
4.));
#35444=CARTESIAN_POINT('Ctrl Pts',(-0.126543984365092,-0.000100563349596846,
3.91934196736194));
#35445=CARTESIAN_POINT('Ctrl Pts',(-0.126601870201444,-0.00676638730964717,
3.91976237798504));
#35446=CARTESIAN_POINT('Ctrl Pts',(-0.126120638953643,-0.0134238307402375,
3.92018278860814));
#35447=CARTESIAN_POINT('Ctrl Pts',(-0.125071086204593,-0.0199904298605203,
3.92060319923124));
#35448=CARTESIAN_POINT('Ctrl Pts',(-0.118463964029756,-0.0613283451774388,
3.92324975925687));
#35449=CARTESIAN_POINT('Ctrl Pts',(-0.089334672430595,-0.0990661662809851,
3.92589631928249));
#35450=CARTESIAN_POINT('Ctrl Pts',(-0.0510182636513927,-0.115928743690777,
3.92854287930812));
#35451=CARTESIAN_POINT('Ctrl Pts',(-0.0127018548721904,-0.132791321100569,
3.93118943933374));
#35452=CARTESIAN_POINT('Ctrl Pts',(0.0348016710870533,-0.128778654816608,
3.93383599935937));
#35453=CARTESIAN_POINT('Ctrl Pts',(0.0697457276620979,-0.10572614363048,
3.93648255938499));
#35454=CARTESIAN_POINT('Ctrl Pts',(0.104689784237142,-0.0826736324443521,
3.93912911941062));
#35455=CARTESIAN_POINT('Ctrl Pts',(0.127074371427988,-0.0405812763560585,
3.94177567943624));
#35456=CARTESIAN_POINT('Ctrl Pts',(0.126652103797309,0.00127848798181101,
3.94442223946187));
#35457=CARTESIAN_POINT('Ctrl Pts',(0.126229836166631,0.0431382523196808,
3.94706879948749));
#35458=CARTESIAN_POINT('Ctrl Pts',(0.103000713714428,0.0847654249071265,
3.94971535951312));
#35459=CARTESIAN_POINT('Ctrl Pts',(0.067598717604338,0.107109484137676,
3.95236191953875));
#35460=CARTESIAN_POINT('Ctrl Pts',(0.0321967214942486,0.129453543368225,
3.95500847956437));
#35461=CARTESIAN_POINT('Ctrl Pts',(-0.0153781482737276,0.132514489241879,
3.95765503958999));
#35462=CARTESIAN_POINT('Ctrl Pts',(-0.0533465659413221,0.114879485769171,
3.96030159961562));
#35463=CARTESIAN_POINT('Ctrl Pts',(-0.0913149836089167,0.0972444822964635,
3.96294815964124));
#35464=CARTESIAN_POINT('Ctrl Pts',(-0.11967694917613,0.0589135294773952,
3.96559471966687));
#35465=CARTESIAN_POINT('Ctrl Pts',(-0.12544884800723,0.0174567123195785,
3.9682412796925));
#35466=CARTESIAN_POINT('Ctrl Pts',(-0.1262490134813,0.0117095024801126,
3.96860817558231));
#35467=CARTESIAN_POINT('Ctrl Pts',(-0.126615029050668,0.00590221784225734,
3.96897507147213));
#35468=CARTESIAN_POINT('Ctrl Pts',(-0.126567406925801,8.9117089303592E-5,
3.96934196736194));
#35469=CARTESIAN_POINT('Ctrl Pts',(-0.0398513841857263,-0.149064942821851,
4.));
#35470=CARTESIAN_POINT('Ctrl Pts',(-0.0894268873061843,-0.13581130730129,
3.99735343997437));
#35471=CARTESIAN_POINT('Ctrl Pts',(-0.173454116750112,-0.0561632816072737,
3.99206031992313));
#35472=CARTESIAN_POINT('Ctrl Pts',(-0.141207051852386,0.115615412698802,
3.98412063984625));
#35473=CARTESIAN_POINT('Ctrl Pts',(0.0205691872966891,0.181176549232701,
3.97618095976937));
#35474=CARTESIAN_POINT('Ctrl Pts',(0.16339053139201,0.0810339956098913,
3.9682412796925));
#35475=CARTESIAN_POINT('Ctrl Pts',(0.156677599794682,-0.0933915431448235,
3.96030159961562));
#35476=CARTESIAN_POINT('Ctrl Pts',(0.00648228676056323,-0.182263829019595,
3.95236191953875));
#35477=CARTESIAN_POINT('Ctrl Pts',(-0.149631704989928,-0.104283093629962,
3.94442223946187));
#35478=CARTESIAN_POINT('Ctrl Pts',(-0.168754687429674,0.0691889583215889,
3.93648255938499));
#35479=CARTESIAN_POINT('Ctrl Pts',(-0.0333654229848094,0.179306981584077,
3.92854287930812));
#35480=CARTESIAN_POINT('Ctrl Pts',(0.132570265831228,0.125258780485074,
3.92060319923124));
#35481=CARTESIAN_POINT('Ctrl Pts',(0.17712875926901,-0.0434751369680033,
3.91266351915436));
#35482=CARTESIAN_POINT('Ctrl Pts',(0.059511610779771,-0.172403375181386,
3.90472383907749));
#35483=CARTESIAN_POINT('Ctrl Pts',(-0.112592720088119,-0.143483428861666,
3.89678415900062));
#35484=CARTESIAN_POINT('Ctrl Pts',(-0.181609867534042,0.0168069012899025,
3.88884447892373));
#35485=CARTESIAN_POINT('Ctrl Pts',(-0.0843490715154628,0.161709102853824,
3.88090479884686));
#35486=CARTESIAN_POINT('Ctrl Pts',(0.0901397770410241,0.158554183500776,
3.87296511876998));
#35487=CARTESIAN_POINT('Ctrl Pts',(0.182098715355847,0.0102306290122647,
3.86502543869311));
#35488=CARTESIAN_POINT('Ctrl Pts',(0.107332199369115,-0.147459841777235,
3.85708575861623));
#35489=CARTESIAN_POINT('Ctrl Pts',(-0.0657052328909015,-0.17013944154474,
3.84914607853936));
#35490=CARTESIAN_POINT('Ctrl Pts',(-0.178584450418103,-0.0370432327022405,
3.84120639846248));
#35491=CARTESIAN_POINT('Ctrl Pts',(-0.127955803747328,0.129968915826709,
3.83326671838561));
#35492=CARTESIAN_POINT('Ctrl Pts',(0.039826267121788,0.177984480821945,
3.82532703830873));
#35493=CARTESIAN_POINT('Ctrl Pts',(0.171144313607041,0.063041501012073,
3.81738735823185));
#35494=CARTESIAN_POINT('Ctrl Pts',(0.145766517224248,-0.109620843643728,
3.80944767815498));
#35495=CARTESIAN_POINT('Ctrl Pts',(-0.0130717883220708,-0.181916836159762,
3.8015079980781));
#35496=CARTESIAN_POINT('Ctrl Pts',(-0.159941861709037,-0.0876539091820477,
3.79356831800123));
#35497=CARTESIAN_POINT('Ctrl Pts',(-0.160372802668024,0.0868629442494614,
3.78562863792435));
#35498=CARTESIAN_POINT('Ctrl Pts',(-0.013970051492431,0.181850060719556,
3.77768895784748));
#35499=CARTESIAN_POINT('Ctrl Pts',(0.145223361235896,0.110339395832533,
3.7697492777706));
#35500=CARTESIAN_POINT('Ctrl Pts',(0.171453565975463,-0.0621955113766863,
3.76180959769372));
#35501=CARTESIAN_POINT('Ctrl Pts',(0.0407047835991549,-0.177785622348059,
3.75386991761685));
#35502=CARTESIAN_POINT('Ctrl Pts',(-0.127312373243651,-0.130599259340906,
3.74593023753997));
#35503=CARTESIAN_POINT('Ctrl Pts',(-0.178765215511242,0.0361608164252855,
3.7379905574631));
#35504=CARTESIAN_POINT('Ctrl Pts',(-0.0665446905722607,0.169812870767156,
3.73005087738622));
#35505=CARTESIAN_POINT('Ctrl Pts',(0.106602640202898,0.147988121222216,
3.72211119730934));
#35506=CARTESIAN_POINT('Ctrl Pts',(0.182147017152552,-0.0093311876933208,
3.71417151723247));
#35507=CARTESIAN_POINT('Ctrl Pts',(0.0909217261957518,-0.158107073301583,
3.70623183715559));
#35508=CARTESIAN_POINT('Ctrl Pts',(-0.0835494302172658,-0.162123717048593,
3.69829215707872));
#35509=CARTESIAN_POINT('Ctrl Pts',(-0.181524627767524,-0.0177035712699219,
3.69035247700185));
#35510=CARTESIAN_POINT('Ctrl Pts',(-0.113300002982309,0.14292556192831,
3.68241279692496));
#35511=CARTESIAN_POINT('Ctrl Pts',(0.0586595287281965,0.172695299861449,
3.67447311684809));
#35512=CARTESIAN_POINT('Ctrl Pts',(0.176911729524118,0.0443491475303153,
3.66653343677121));
#35513=CARTESIAN_POINT('Ctrl Pts',(0.133187572742707,-0.124602076359984,
3.65859375669434));
#35514=CARTESIAN_POINT('Ctrl Pts',(-0.0324800977009374,-0.179470471240069,
3.65065407661746));
#35515=CARTESIAN_POINT('Ctrl Pts',(-0.168409729113823,-0.0700197840611982,
3.64271439654059));
#35516=CARTESIAN_POINT('Ctrl Pts',(-0.150147241221285,0.103539428007117,
3.63477471646371));
#35517=CARTESIAN_POINT('Ctrl Pts',(0.00558664719359638,0.182300288895857,
3.62683503638684));
#35518=CARTESIAN_POINT('Ctrl Pts',(0.156205528517827,0.094151159125646,
3.61889535630996));
#35519=CARTESIAN_POINT('Ctrl Pts',(0.163806179027695,-0.0802006497663837,
3.61095567623308));
#35520=CARTESIAN_POINT('Ctrl Pts',(0.0214296163208854,-0.181122531330724,
3.60301599615621));
#35521=CARTESIAN_POINT('Ctrl Pts',(-0.140567416427732,-0.116212810634341,
3.59507631607934));
#35522=CARTESIAN_POINT('Ctrl Pts',(-0.173864117377934,0.0550988535555318,
3.58713663600245));
#35523=CARTESIAN_POINT('Ctrl Pts',(-0.0479747871584019,0.175962994372803,
3.57919695592558));
#35524=CARTESIAN_POINT('Ctrl Pts',(0.121839171429706,0.13571993663382,3.5712572758487));
#35525=CARTESIAN_POINT('Ctrl Pts',(0.180099946935509,-0.0287862221383337,
3.56331759577183));
#35526=CARTESIAN_POINT('Ctrl Pts',(0.0734653204375665,-0.166934393666355,
3.55537791569495));
#35527=CARTESIAN_POINT('Ctrl Pts',(-0.100432512451176,-0.152245088347237,
3.54743823561807));
#35528=CARTESIAN_POINT('Ctrl Pts',(-0.182376563237206,0.00184389181179004,
3.5394985555412));
#35529=CARTESIAN_POINT('Ctrl Pts',(-0.0973408901199132,0.154229940417525,
3.53155887546432));
#35530=CARTESIAN_POINT('Ctrl Pts',(0.0768181056158631,0.16543527210962,
3.52361919538745));
#35531=CARTESIAN_POINT('Ctrl Pts',(0.180643771975638,0.0251157687415861,
3.51567951531057));
#35532=CARTESIAN_POINT('Ctrl Pts',(0.11907687582224,-0.13808957637103,3.50773983523369));
#35533=CARTESIAN_POINT('Ctrl Pts',(-0.0515150906951779,-0.17507869823889,
3.49980015515682));
#35534=CARTESIAN_POINT('Ctrl Pts',(-0.174944455635001,-0.0513330523253054,
3.49186047507995));
#35535=CARTESIAN_POINT('Ctrl Pts',(-0.15040278985559,0.061813268541742,
3.4865673550287));
#35536=CARTESIAN_POINT('Ctrl Pts',(-0.116913659442529,0.100696009035892,
3.48392079500307));
#35537=CARTESIAN_POINT('Ctrl Pts',(-0.0374537582415214,-0.140096572423085,
4.00535973499898));
#35538=CARTESIAN_POINT('Ctrl Pts',(-0.0840465917531983,-0.127640331046503,
4.00271317497335));
#35539=CARTESIAN_POINT('Ctrl Pts',(-0.163018391644278,-0.0527842636924701,
3.9974200549221));
#35540=CARTESIAN_POINT('Ctrl Pts',(-0.132711445038627,0.108659505929172,
3.98948037484522));
#35541=CARTESIAN_POINT('Ctrl Pts',(0.0193316589618159,0.170276210290963,
3.98154069476835));
#35542=CARTESIAN_POINT('Ctrl Pts',(0.153560273670542,0.0761586515231869,
3.97360101469147));
#35543=CARTESIAN_POINT('Ctrl Pts',(0.147251220113796,-0.0877727173150906,
3.9656613346146));
#35544=CARTESIAN_POINT('Ctrl Pts',(0.00609228527799324,-0.171298074778515,
3.95772165453772));
#35545=CARTESIAN_POINT('Ctrl Pts',(-0.140629235808745,-0.0980089865709976,
3.94978197446085));
#35546=CARTESIAN_POINT('Ctrl Pts',(-0.158601699646316,0.0650262612179893,
3.94184229438397));
#35547=CARTESIAN_POINT('Ctrl Pts',(-0.0313580195928739,0.168519123651227,
3.93390261430709));
#35548=CARTESIAN_POINT('Ctrl Pts',(0.124594284186381,0.117722688377688,
3.92596293423022));
#35549=CARTESIAN_POINT('Ctrl Pts',(0.166471952300676,-0.0408594909006909,
3.91802325415334));
#35550=CARTESIAN_POINT('Ctrl Pts',(0.0559311433781364,-0.162030867082874,
3.91008357407647));
#35551=CARTESIAN_POINT('Ctrl Pts',(-0.105818671147842,-0.134850865686472,
3.90214389399959));
#35552=CARTESIAN_POINT('Ctrl Pts',(-0.170683458351015,0.0157957278163147,
3.89420421392272));
#35553=CARTESIAN_POINT('Ctrl Pts',(-0.0792742785975418,0.151980006905501,
3.88626453384583));
#35554=CARTESIAN_POINT('Ctrl Pts',(0.0847165910600508,0.149014900695642,
3.87832485376897));
#35555=CARTESIAN_POINT('Ctrl Pts',(0.171142895043338,0.00961511158303258,
3.87038517369209));
#35556=CARTESIAN_POINT('Ctrl Pts',(0.100874645356521,-0.138588040970374,
3.86244549361521));
#35557=CARTESIAN_POINT('Ctrl Pts',(-0.0617521312792973,-0.159903141162322,
3.85450581353833));
#35558=CARTESIAN_POINT('Ctrl Pts',(-0.16784006298206,-0.0348145568958948,
3.84656613346146));
#35559=CARTESIAN_POINT('Ctrl Pts',(-0.120257447440646,0.122149442277835,
3.83862645338458));
#35560=CARTESIAN_POINT('Ctrl Pts',(0.0374301523251976,0.167276190066077,
3.83068677330771));
#35561=CARTESIAN_POINT('Ctrl Pts',(0.16084755591865,0.0592486606509017,
3.82274709323083));
#35562=CARTESIAN_POINT('Ctrl Pts',(0.136996593904535,-0.103025595219711,
3.81480741315396));
#35563=CARTESIAN_POINT('Ctrl Pts',(-0.0122853348660984,-0.170971958460368,
3.80686773307708));
#35564=CARTESIAN_POINT('Ctrl Pts',(-0.150319090379167,-0.0823802834081873,
3.7989280530002));
#35565=CARTESIAN_POINT('Ctrl Pts',(-0.150724104127725,0.0816369062340208,
3.79098837292333));
#35566=CARTESIAN_POINT('Ctrl Pts',(-0.0131295547672976,0.170909200509922,
3.78304869284645));
#35567=CARTESIAN_POINT('Ctrl Pts',(0.136486116452099,0.103700916303616,
3.77510901276958));
#35568=CARTESIAN_POINT('Ctrl Pts',(0.161138202371193,-0.0584535692901865,
3.7671693326927));
#35569=CARTESIAN_POINT('Ctrl Pts',(0.0382558135770412,-0.167089295749672,
3.75922965261583));
#35570=CARTESIAN_POINT('Ctrl Pts',(-0.119652728407108,-0.122741861689914,
3.75128997253895));
#35571=CARTESIAN_POINT('Ctrl Pts',(-0.168009952491177,0.0339852304727166,
3.74335029246208));
#35572=CARTESIAN_POINT('Ctrl Pts',(-0.0625410836756577,0.159596218248545,
3.73541061238519));
#35573=CARTESIAN_POINT('Ctrl Pts',(0.100188979521,0.139084536914507,3.72747093230832));
#35574=CARTESIAN_POINT('Ctrl Pts',(0.171188290801939,-0.00876978441559563,
3.71953125223144));
#35575=CARTESIAN_POINT('Ctrl Pts',(0.0854514948832616,-0.148594690515994,
3.71159157215457));
#35576=CARTESIAN_POINT('Ctrl Pts',(-0.078522747064207,-0.15236967617626,
3.7036518920777));
#35577=CARTESIAN_POINT('Ctrl Pts',(-0.170603346965352,-0.0166384503801673,
3.69571221200081));
#35578=CARTESIAN_POINT('Ctrl Pts',(-0.106483400945028,0.134326562361009,
3.68777253192394));
#35579=CARTESIAN_POINT('Ctrl Pts',(0.0551303261464719,0.162305228353258,
3.67983285184707));
#35580=CARTESIAN_POINT('Ctrl Pts',(0.166267979972926,0.0416809173321745,
3.67189317177019));
#35581=CARTESIAN_POINT('Ctrl Pts',(0.125174451332285,-0.117105494319316,
3.66395349169331));
#35582=CARTESIAN_POINT('Ctrl Pts',(-0.030525959180801,-0.168672777085747,
3.65601381161644));
#35583=CARTESIAN_POINT('Ctrl Pts',(-0.158277495465476,-0.0658071010063173,
3.64807413153956));
#35584=CARTESIAN_POINT('Ctrl Pts',(-0.141113755224281,0.0973100629822772,
3.64013445146269));
#35585=CARTESIAN_POINT('Ctrl Pts',(0.0052505311332342,0.171332341076135,
3.63219477138581));
#35586=CARTESIAN_POINT('Ctrl Pts',(0.146807550619315,0.0884866316215429,
3.62425509130893));
#35587=CARTESIAN_POINT('Ctrl Pts',(0.153950914206089,-0.0753754432509509,
3.61631541123206));
#35588=CARTESIAN_POINT('Ctrl Pts',(0.0201403209773194,-0.170225442331889,
3.60837573115518));
#35589=CARTESIAN_POINT('Ctrl Pts',(-0.132110292756286,-0.109220961906395,
3.60043605107832));
#35590=CARTESIAN_POINT('Ctrl Pts',(-0.163403724919573,0.0517838760841091,
3.59249637100142));
#35591=CARTESIAN_POINT('Ctrl Pts',(-0.0450884233166185,0.165376324696236,
3.58455669092456));
#35592=CARTESIAN_POINT('Ctrl Pts',(0.114508817305019,0.12755445762053,3.57661701084768));
#35593=CARTESIAN_POINT('Ctrl Pts',(0.169264380890674,-0.0270543226210457,
3.56867733077081));
#35594=CARTESIAN_POINT('Ctrl Pts',(0.0690453395039173,-0.156890922368865,
3.56073765069393));
#35595=CARTESIAN_POINT('Ctrl Pts',(-0.0943900724603247,-0.14308538709325,
3.55279797061705));
#35596=CARTESIAN_POINT('Ctrl Pts',(-0.171404026434103,0.00173295556863096,
3.54485829054018));
#35597=CARTESIAN_POINT('Ctrl Pts',(-0.0914844550586914,0.144950822161685,
3.5369186104633));
#35598=CARTESIAN_POINT('Ctrl Pts',(0.0721964071034376,0.155481994234803,
3.52897893038643));
#35599=CARTESIAN_POINT('Ctrl Pts',(0.169775487141934,0.0236046990516893,
3.52103925030955));
#35600=CARTESIAN_POINT('Ctrl Pts',(0.111912712954128,-0.129781529920537,
3.51309957023267));
#35601=CARTESIAN_POINT('Ctrl Pts',(-0.0484157273859087,-0.164545231516157,
3.5051598901558));
#35602=CARTESIAN_POINT('Ctrl Pts',(-0.164419065508765,-0.0482446412057121,
3.49722021007893));
#35603=CARTESIAN_POINT('Ctrl Pts',(-0.141353928983959,0.0580943237828579,
3.49192709002767));
#35604=CARTESIAN_POINT('Ctrl Pts',(-0.109879644719102,0.094637715988474,
3.48928053000205));
#35605=CARTESIAN_POINT('Ctrl Pts',(-0.0350561322973164,-0.13112820202432,
4.01071946999795));
#35606=CARTESIAN_POINT('Ctrl Pts',(-0.0786662962002123,-0.119469354791716,
4.00807290997233));
#35607=CARTESIAN_POINT('Ctrl Pts',(-0.152582666538444,-0.0494052457776665,
4.00277978992108));
#35608=CARTESIAN_POINT('Ctrl Pts',(-0.124215838224868,0.101703599159542,
3.9948401098442));
#35609=CARTESIAN_POINT('Ctrl Pts',(0.0180941306269427,0.159375871349225,
3.98690042976732));
#35610=CARTESIAN_POINT('Ctrl Pts',(0.143730015949074,0.0712833074364824,
3.97896074969045));
#35611=CARTESIAN_POINT('Ctrl Pts',(0.137824840432911,-0.0821538914853577,
3.97102106961357));
#35612=CARTESIAN_POINT('Ctrl Pts',(0.0057022837954231,-0.160332320537436,
3.9630813895367));
#35613=CARTESIAN_POINT('Ctrl Pts',(-0.131626766627563,-0.0917348795120337,
3.95514170945982));
#35614=CARTESIAN_POINT('Ctrl Pts',(-0.148448711862958,0.0608635641143897,
3.94720202938295));
#35615=CARTESIAN_POINT('Ctrl Pts',(-0.0293506162009384,0.157731265718376,
3.93926234930607));
#35616=CARTESIAN_POINT('Ctrl Pts',(0.116618302541534,0.110186596270301,
3.93132266922919));
#35617=CARTESIAN_POINT('Ctrl Pts',(0.155815145332341,-0.0382438448333786,
3.92338298915232));
#35618=CARTESIAN_POINT('Ctrl Pts',(0.0523506759765019,-0.151658358984361,
3.91544330907544));
#35619=CARTESIAN_POINT('Ctrl Pts',(-0.0990446222075651,-0.126218302511277,
3.90750362899857));
#35620=CARTESIAN_POINT('Ctrl Pts',(-0.159757049167988,0.0147845543427269,
3.89956394892169));
#35621=CARTESIAN_POINT('Ctrl Pts',(-0.0741994856796208,0.142250910957177,
3.89162426884482));
#35622=CARTESIAN_POINT('Ctrl Pts',(0.0792934050790776,0.139475617890508,
3.88368458876794));
#35623=CARTESIAN_POINT('Ctrl Pts',(0.160187074730829,0.0089995941538004,
3.87574490869107));
#35624=CARTESIAN_POINT('Ctrl Pts',(0.0944170913439271,-0.129716240163513,
3.86780522861419));
#35625=CARTESIAN_POINT('Ctrl Pts',(-0.0577990296676931,-0.149666840779905,
3.85986554853731));
#35626=CARTESIAN_POINT('Ctrl Pts',(-0.157095675546018,-0.0325858810895492,
3.85192586846044));
#35627=CARTESIAN_POINT('Ctrl Pts',(-0.112559091133964,0.114329968728961,
3.84398618838356));
#35628=CARTESIAN_POINT('Ctrl Pts',(0.0350340375286068,0.156567899310209,
3.83604650830669));
#35629=CARTESIAN_POINT('Ctrl Pts',(0.150550798230259,0.0554558202897304,
3.8281068282298));
#35630=CARTESIAN_POINT('Ctrl Pts',(0.128226670584821,-0.0964303467956928,
3.82016714815294));
#35631=CARTESIAN_POINT('Ctrl Pts',(-0.0114988814101258,-0.160027080760974,
3.81222746807605));
#35632=CARTESIAN_POINT('Ctrl Pts',(-0.140696319049298,-0.0771066576343268,
3.80428778799918));
#35633=CARTESIAN_POINT('Ctrl Pts',(-0.141075405587426,0.0764108682185801,
3.79634810792231));
#35634=CARTESIAN_POINT('Ctrl Pts',(-0.0122890580421644,0.159968340300288,
3.78840842784543));
#35635=CARTESIAN_POINT('Ctrl Pts',(0.127748871668302,0.0970624367746977,
3.78046874776856));
#35636=CARTESIAN_POINT('Ctrl Pts',(0.150822838766923,-0.0547116272036868,
3.77252906769167));
#35637=CARTESIAN_POINT('Ctrl Pts',(0.0358068435549273,-0.156392969151285,
3.7645893876148));
#35638=CARTESIAN_POINT('Ctrl Pts',(-0.111993083570565,-0.114884464038922,
3.75664970753792));
#35639=CARTESIAN_POINT('Ctrl Pts',(-0.157254689471112,0.0318096445201475,
3.74871002746105));
#35640=CARTESIAN_POINT('Ctrl Pts',(-0.0585374767790549,0.149379565729933,
3.74077034738417));
#35641=CARTESIAN_POINT('Ctrl Pts',(0.0937753188391016,0.130180952606797,
3.7328306673073));
#35642=CARTESIAN_POINT('Ctrl Pts',(0.160229564451327,-0.00820838113787044,
3.72489098723042));
#35643=CARTESIAN_POINT('Ctrl Pts',(0.0799812635707716,-0.139082307730405,
3.71695130715355));
#35644=CARTESIAN_POINT('Ctrl Pts',(-0.0734960639111485,-0.142615635303926,
3.70901162707667));
#35645=CARTESIAN_POINT('Ctrl Pts',(-0.15968206616318,-0.015573329490413,
3.7010719469998));
#35646=CARTESIAN_POINT('Ctrl Pts',(-0.0996667989077476,0.125727562793709,
3.69313226692292));
#35647=CARTESIAN_POINT('Ctrl Pts',(0.0516011235647474,0.151915156845068,
3.68519258684604));
#35648=CARTESIAN_POINT('Ctrl Pts',(0.155624230421734,0.039012687134034,
3.67725290676917));
#35649=CARTESIAN_POINT('Ctrl Pts',(0.117161329921862,-0.109608912278647,
3.66931322669229));
#35650=CARTESIAN_POINT('Ctrl Pts',(-0.0285718206606646,-0.157875082931424,
3.66137354661541));
#35651=CARTESIAN_POINT('Ctrl Pts',(-0.148145261817129,-0.0615944179514364,
3.65343386653854));
#35652=CARTESIAN_POINT('Ctrl Pts',(-0.132080269227278,0.0910806979574378,
3.64549418646166));
#35653=CARTESIAN_POINT('Ctrl Pts',(0.00491441507287188,0.160364393256412,
3.63755450638479));
#35654=CARTESIAN_POINT('Ctrl Pts',(0.137409572720802,0.08282210411744,3.62961482630791));
#35655=CARTESIAN_POINT('Ctrl Pts',(0.144095649384483,-0.0705502367355182,
3.62167514623104));
#35656=CARTESIAN_POINT('Ctrl Pts',(0.0188510256337537,-0.159328353333054,
3.61373546615416));
#35657=CARTESIAN_POINT('Ctrl Pts',(-0.12365316908484,-0.102229113178448,
3.60579578607729));
#35658=CARTESIAN_POINT('Ctrl Pts',(-0.152943332461211,0.0484688986126864,
3.5978561060004));
#35659=CARTESIAN_POINT('Ctrl Pts',(-0.0422020594748354,0.15478965501967,
3.58991642592354));
#35660=CARTESIAN_POINT('Ctrl Pts',(0.107178463180333,0.119388978607241,
3.58197674584666));
#35661=CARTESIAN_POINT('Ctrl Pts',(0.15842881484584,-0.0253224231037578,
3.57403706576978));
#35662=CARTESIAN_POINT('Ctrl Pts',(0.0646253585702682,-0.146847451071376,
3.56609738569291));
#35663=CARTESIAN_POINT('Ctrl Pts',(-0.0883476324694729,-0.133925685839263,
3.55815770561603));
#35664=CARTESIAN_POINT('Ctrl Pts',(-0.160431489631001,0.00162201932547174,
3.55021802553915));
#35665=CARTESIAN_POINT('Ctrl Pts',(-0.0856280199974695,0.135671703905846,
3.54227834546228));
#35666=CARTESIAN_POINT('Ctrl Pts',(0.067574708591012,0.145528716359985,
3.5343386653854));
#35667=CARTESIAN_POINT('Ctrl Pts',(0.15890720230823,0.0220936293617927,
3.52639898530853));
#35668=CARTESIAN_POINT('Ctrl Pts',(0.104748550086015,-0.121473483470044,
3.51845930523165));
#35669=CARTESIAN_POINT('Ctrl Pts',(-0.0453163640766394,-0.154011764793424,
3.51051962515478));
#35670=CARTESIAN_POINT('Ctrl Pts',(-0.153893675382528,-0.0451562300861186,
3.5025799450779));
#35671=CARTESIAN_POINT('Ctrl Pts',(-0.132305068112328,0.0543753790239735,
3.49728682502665));
#35672=CARTESIAN_POINT('Ctrl Pts',(-0.102845629995675,0.0885794229410565,
3.49464026500102));
#35673=CARTESIAN_POINT('Ctrl Pts',(-0.0326585063531114,-0.122159831625554,
4.01607920499693));
#35674=CARTESIAN_POINT('Ctrl Pts',(-0.0732860006472263,-0.111298378536929,
4.0134326449713));
#35675=CARTESIAN_POINT('Ctrl Pts',(-0.142146941432609,-0.046026227862863,
4.00813952492006));
#35676=CARTESIAN_POINT('Ctrl Pts',(-0.11572023141111,0.0947476923899126,
4.00019984484318));
#35677=CARTESIAN_POINT('Ctrl Pts',(0.0168566022920696,0.148475532407486,
3.9922601647663));
#35678=CARTESIAN_POINT('Ctrl Pts',(0.133899758227606,0.0664079633497781,
3.98432048468943));
#35679=CARTESIAN_POINT('Ctrl Pts',(0.128398460752025,-0.076535065655625,
3.97638080461255));
#35680=CARTESIAN_POINT('Ctrl Pts',(0.00531228231285306,-0.149366566296356,
3.96844112453568));
#35681=CARTESIAN_POINT('Ctrl Pts',(-0.12262429744638,-0.0854607724530698,
3.9605014444588));
#35682=CARTESIAN_POINT('Ctrl Pts',(-0.1382957240796,0.0567008670107902,
3.95256176438192));
#35683=CARTESIAN_POINT('Ctrl Pts',(-0.0273432128090029,0.146943407785525,
3.94462208430505));
#35684=CARTESIAN_POINT('Ctrl Pts',(0.108642320896687,0.102650504162914,
3.93668240422817));
#35685=CARTESIAN_POINT('Ctrl Pts',(0.145158338364007,-0.0356281987660663,
3.9287427241513));
#35686=CARTESIAN_POINT('Ctrl Pts',(0.0487702085748674,-0.141285850885848,
3.92080304407442));
#35687=CARTESIAN_POINT('Ctrl Pts',(-0.0922705732672884,-0.117585739336083,
3.91286336399754));
#35688=CARTESIAN_POINT('Ctrl Pts',(-0.148830639984962,0.0137733808691391,
3.90492368392067));
#35689=CARTESIAN_POINT('Ctrl Pts',(-0.0691246927616998,0.132521815008853,
3.89698400384379));
#35690=CARTESIAN_POINT('Ctrl Pts',(0.0738702190981043,0.129936335085374,
3.88904432376692));
#35691=CARTESIAN_POINT('Ctrl Pts',(0.149231254418321,0.00838407672456824,
3.88110464369004));
#35692=CARTESIAN_POINT('Ctrl Pts',(0.0879595373313327,-0.120844439356652,
3.87316496361317));
#35693=CARTESIAN_POINT('Ctrl Pts',(-0.0538459280560888,-0.139430540397488,
3.86522528353628));
#35694=CARTESIAN_POINT('Ctrl Pts',(-0.146351288109975,-0.0303572052832036,
3.85728560345941));
#35695=CARTESIAN_POINT('Ctrl Pts',(-0.104860734827282,0.106510495180087,
3.84934592338253));
#35696=CARTESIAN_POINT('Ctrl Pts',(0.0326379227320163,0.145859608554342,
3.84140624330567));
#35697=CARTESIAN_POINT('Ctrl Pts',(0.140254040541868,0.0516629799285589,
3.83346656322878));
#35698=CARTESIAN_POINT('Ctrl Pts',(0.119456747265108,-0.0898350983716749,
3.82552688315191));
#35699=CARTESIAN_POINT('Ctrl Pts',(-0.0107124279541533,-0.14908220306158,
3.81758720307504));
#35700=CARTESIAN_POINT('Ctrl Pts',(-0.131073547719428,-0.0718330318604663,
3.80964752299816));
#35701=CARTESIAN_POINT('Ctrl Pts',(-0.131426707047127,0.0711848302031395,
3.80170784292129));
#35702=CARTESIAN_POINT('Ctrl Pts',(-0.0114485613170311,0.149027480090653,
3.7937681628444));
#35703=CARTESIAN_POINT('Ctrl Pts',(0.119011626884504,0.0904239572457801,
3.78582848276753));
#35704=CARTESIAN_POINT('Ctrl Pts',(0.140507475162653,-0.0509696851171873,
3.77788880269065));
#35705=CARTESIAN_POINT('Ctrl Pts',(0.0333578735328136,-0.145696642552897,
3.76994912261378));
#35706=CARTESIAN_POINT('Ctrl Pts',(-0.104333438734023,-0.10702706638793,
3.7620094425369));
#35707=CARTESIAN_POINT('Ctrl Pts',(-0.146499426451047,0.0296340585675785,
3.75406976246003));
#35708=CARTESIAN_POINT('Ctrl Pts',(-0.0545338698824522,0.139162913211322,
3.74613008238315));
#35709=CARTESIAN_POINT('Ctrl Pts',(0.0873616581572035,0.121277368299088,
3.73819040230628));
#35710=CARTESIAN_POINT('Ctrl Pts',(0.149270838100714,-0.00764697786014525,
3.7302507222294));
#35711=CARTESIAN_POINT('Ctrl Pts',(0.0745110322582815,-0.129569924944816,
3.72231104215252));
#35712=CARTESIAN_POINT('Ctrl Pts',(-0.0684693807580898,-0.132861594431592,
3.71437136207565));
#35713=CARTESIAN_POINT('Ctrl Pts',(-0.148760785361007,-0.0145082086006585,
3.70643168199877));
#35714=CARTESIAN_POINT('Ctrl Pts',(-0.0928501968704667,0.117128563226408,
3.6984920019219));
#35715=CARTESIAN_POINT('Ctrl Pts',(0.0480719209830229,0.141525085336877,
3.69055232184502));
#35716=CARTESIAN_POINT('Ctrl Pts',(0.144980480870543,0.0363444569358934,
3.68261264176815));
#35717=CARTESIAN_POINT('Ctrl Pts',(0.10914820851144,-0.102112330237978,
3.67467296169127));
#35718=CARTESIAN_POINT('Ctrl Pts',(-0.0266176821405283,-0.147077388777102,
3.66673328161439));
#35719=CARTESIAN_POINT('Ctrl Pts',(-0.138013028168781,-0.0573817348965553,
3.65879360153751));
#35720=CARTESIAN_POINT('Ctrl Pts',(-0.123046783230275,0.0848513329325982,
3.65085392146064));
#35721=CARTESIAN_POINT('Ctrl Pts',(0.00457829901250977,0.149396445436689,
3.64291424138376));
#35722=CARTESIAN_POINT('Ctrl Pts',(0.128011594822289,0.0771575766133371,
3.63497456130689));
#35723=CARTESIAN_POINT('Ctrl Pts',(0.134240384562878,-0.0657250302200856,
3.62703488123001));
#35724=CARTESIAN_POINT('Ctrl Pts',(0.0175617302901878,-0.148431264334219,
3.61909520115314));
#35725=CARTESIAN_POINT('Ctrl Pts',(-0.115196045413394,-0.0952372644505018,
3.61115552107626));
#35726=CARTESIAN_POINT('Ctrl Pts',(-0.14248294000285,0.0451539211412638,
3.60321584099938));
#35727=CARTESIAN_POINT('Ctrl Pts',(-0.039315695633052,0.144202985343104,
3.59527616092251));
#35728=CARTESIAN_POINT('Ctrl Pts',(0.0998481090556468,0.111223499593951,
3.58733648084563));
#35729=CARTESIAN_POINT('Ctrl Pts',(0.147593248801005,-0.0235905235864699,
3.57939680076876));
#35730=CARTESIAN_POINT('Ctrl Pts',(0.0602053776366188,-0.136803979773886,
3.57145712069188));
#35731=CARTESIAN_POINT('Ctrl Pts',(-0.0823051924786211,-0.124765984585276,
3.56351744061501));
#35732=CARTESIAN_POINT('Ctrl Pts',(-0.149458952827898,0.00151108308231263,
3.55557776053813));
#35733=CARTESIAN_POINT('Ctrl Pts',(-0.0797715849362477,0.126392585650007,
3.54763808046126));
#35734=CARTESIAN_POINT('Ctrl Pts',(0.0629530100785864,0.135575438485168,
3.53969840038438));
#35735=CARTESIAN_POINT('Ctrl Pts',(0.148038917474527,0.020582559671896,
3.5317587203075));
#35736=CARTESIAN_POINT('Ctrl Pts',(0.097584387217902,-0.113165437019551,
3.52381904023062));
#35737=CARTESIAN_POINT('Ctrl Pts',(-0.0422170007673702,-0.143478298070691,
3.51587936015375));
#35738=CARTESIAN_POINT('Ctrl Pts',(-0.143368285256292,-0.0420678189665254,
3.50793968007687));
#35739=CARTESIAN_POINT('Ctrl Pts',(-0.123256207240696,0.0506564342650893,
3.50264656002563));
#35740=CARTESIAN_POINT('Ctrl Pts',(-0.0958116152722475,0.0825211298936389,
3.5));
#35741=CARTESIAN_POINT('Ctrl Pts',(-0.126283770505697,7.06948412972308E-5,
3.95565803263806));
#35742=CARTESIAN_POINT('Ctrl Pts',(-0.126367959766412,0.0165211867142232,
3.95462594321935));
#35743=CARTESIAN_POINT('Ctrl Pts',(-0.123384590961307,0.0329424219101817,
3.95359385380063));
#35744=CARTESIAN_POINT('Ctrl Pts',(-0.117191734428964,0.0480476838959361,
3.95256176438192));
#35745=CARTESIAN_POINT('Ctrl Pts',(-0.101311553656068,0.086781713935702,
3.9499152043563));
#35746=CARTESIAN_POINT('Ctrl Pts',(-0.0643273832325353,0.116862560860614,
3.94726864433067));
#35747=CARTESIAN_POINT('Ctrl Pts',(-0.0231710424031541,0.124520833719301,
3.94462208430505));
#35748=CARTESIAN_POINT('Ctrl Pts',(0.0179852984262271,0.132179106577988,
3.94197552427942));
#35749=CARTESIAN_POINT('Ctrl Pts',(0.0633138096614572,0.117414805370451,
3.9393289642538));
#35750=CARTESIAN_POINT('Ctrl Pts',(0.0920640681902922,0.0869862042785193,
3.93668240422817));
#35751=CARTESIAN_POINT('Ctrl Pts',(0.120814326719127,0.0565576031865874,
3.93403584420254));
#35752=CARTESIAN_POINT('Ctrl Pts',(0.132986332541567,0.0104647022102606,
3.93138928417692));
#35753=CARTESIAN_POINT('Ctrl Pts',(0.123007647154597,-0.0301913569645331,
3.9287427241513));
#35754=CARTESIAN_POINT('Ctrl Pts',(0.113028961767627,-0.0708474161393267,
3.92609616412567));
#35755=CARTESIAN_POINT('Ctrl Pts',(0.0808995851712473,-0.106066633512587,
3.92344960410005));
#35756=CARTESIAN_POINT('Ctrl Pts',(0.0413280998993647,-0.11972622360759,
3.92080304407442));
#35757=CARTESIAN_POINT('Ctrl Pts',(0.00175661462748208,-0.133385813702593,
3.91815648404879));
#35758=CARTESIAN_POINT('Ctrl Pts',(-0.0452569793199031,-0.125485776519338,
3.91550992402317));
#35759=CARTESIAN_POINT('Ctrl Pts',(-0.0781904540798746,-0.0996425712268402,
3.91286336399754));
#35760=CARTESIAN_POINT('Ctrl Pts',(-0.10807787979064,-0.0761896290779491,
3.91046158687771));
#35761=CARTESIAN_POINT('Ctrl Pts',(-0.126369304595299,-0.037959184630699,
3.90805980975789));
#35762=CARTESIAN_POINT('Ctrl Pts',(-0.126614009842867,6.71750503076223E-5,
3.90565803263806));
#35763=CARTESIAN_POINT('Ctrl Pts',(-0.0398513841857263,-0.149064942821851,
4.));
#35764=CARTESIAN_POINT('Ctrl Pts',(-0.0498814023543805,-0.14540001546545,
4.));
#35765=CARTESIAN_POINT('Ctrl Pts',(-0.0594354697797451,-0.140634945951871,
4.));
#35766=CARTESIAN_POINT('Ctrl Pts',(-0.0684028880593604,-0.13492060142061,
4.));
#35767=CARTESIAN_POINT('Ctrl Pts',(-0.0752795449518356,-0.130538561296954,
4.));
#35768=CARTESIAN_POINT('Ctrl Pts',(-0.0818109545260972,-0.125596962852027,
4.));
#35769=CARTESIAN_POINT('Ctrl Pts',(-0.0879325986341956,-0.120150358192012,
4.));
#35770=CARTESIAN_POINT('Ctrl Pts',(-0.0903223739843738,-0.118024105615282,
4.));
#35771=CARTESIAN_POINT('Ctrl Pts',(-0.0926479810229214,-0.115821878910758,
4.));
#35772=CARTESIAN_POINT('Ctrl Pts',(-0.0948977224364798,-0.11355536832373,
4.));
#35773=CARTESIAN_POINT('Ctrl Pts',(-0.1022475948872,-0.106150711227375,
4.));
#35774=CARTESIAN_POINT('Ctrl Pts',(-0.108817076574654,-0.0980392058992304,
4.));
#35775=CARTESIAN_POINT('Ctrl Pts',(-0.114476228961537,-0.0893439955398699,
4.));
#35776=CARTESIAN_POINT('Ctrl Pts',(-0.117310911144628,-0.0849885450768213,
4.));
#35777=CARTESIAN_POINT('Ctrl Pts',(-0.119916487835761,-0.0804862654238585,
4.));
#35778=CARTESIAN_POINT('Ctrl Pts',(-0.122271719969265,-0.0758513570938915,
4.));
#35779=CARTESIAN_POINT('Ctrl Pts',(-0.123706258421051,-0.073028300238791,
4.));
#35780=CARTESIAN_POINT('Ctrl Pts',(-0.12504717142243,-0.0701567413128179,
4.));
#35781=CARTESIAN_POINT('Ctrl Pts',(-0.126284991686486,-0.067251866211871,
4.));
#35782=CARTESIAN_POINT('Ctrl Pts',(-0.1295973650463,-0.0594784994498528,
4.));
#35783=CARTESIAN_POINT('Ctrl Pts',(-0.132185052379765,-0.051445045564302,
4.));
#35784=CARTESIAN_POINT('Ctrl Pts',(-0.133964990884521,-0.0432169428549209,
4.));
#35785=CARTESIAN_POINT('Ctrl Pts',(-0.135518726559135,-0.0360345055517295,
4.));
#35786=CARTESIAN_POINT('Ctrl Pts',(-0.13645631947854,-0.0287032207927444,
4.));
#35787=CARTESIAN_POINT('Ctrl Pts',(-0.136789702571871,-0.0212983790736885,
4.));
#35788=CARTESIAN_POINT('Ctrl Pts',(-0.13693233353465,-0.0181303728827948,
4.));
#35789=CARTESIAN_POINT('Ctrl Pts',(-0.136963744111631,-0.0149584576035291,
4.));
#35790=CARTESIAN_POINT('Ctrl Pts',(-0.136886254945713,-0.0117904221806244,
4.));
#35791=CARTESIAN_POINT('Ctrl Pts',(-0.136677592311597,-0.00325954423806801,
4.));
#35792=CARTESIAN_POINT('Ctrl Pts',(-0.135681410366555,0.00524856144622462,
4.));
#35793=CARTESIAN_POINT('Ctrl Pts',(-0.133925248777689,0.0136159175851835,
4.));
#35794=CARTESIAN_POINT('Ctrl Pts',(-0.132934632228228,0.018335780221422,
4.));
#35795=CARTESIAN_POINT('Ctrl Pts',(-0.131701699385377,0.0230107212566983,
4.));
#35796=CARTESIAN_POINT('Ctrl Pts',(-0.130227956640556,0.0276173752808998,
4.));
#35797=CARTESIAN_POINT('Ctrl Pts',(-0.129158656751422,0.030959813881302,
4.));
#35798=CARTESIAN_POINT('Ctrl Pts',(-0.12796229886657,0.0342658696738965,
4.));
#35799=CARTESIAN_POINT('Ctrl Pts',(-0.126644858507038,0.0375136883583919,
4.));
#35800=CARTESIAN_POINT('Ctrl Pts',(-0.124572648602295,0.042622201998594,
4.));
#35801=CARTESIAN_POINT('Ctrl Pts',(-0.122198572282107,0.0475953519381505,
4.));
#35802=CARTESIAN_POINT('Ctrl Pts',(-0.119526530046339,0.0523977893098404,
4.));
#35803=CARTESIAN_POINT('Ctrl Pts',(-0.116935312520942,0.0570549611597328,
4.));
#35804=CARTESIAN_POINT('Ctrl Pts',(-0.11406058633243,0.0615550019486321,
4.));
#35805=CARTESIAN_POINT('Ctrl Pts',(-0.11092106856286,0.0658392337664117,
4.));
#35806=CARTESIAN_POINT('Ctrl Pts',(-0.10710607669906,0.071045227402084,
4.));
#35807=CARTESIAN_POINT('Ctrl Pts',(-0.102897192277319,0.075940267594365,
4.));
#35808=CARTESIAN_POINT('Ctrl Pts',(-0.0982968852906839,0.0804596595786888,
4.));
#35809=CARTESIAN_POINT('Ctrl Pts',(-0.0975398380300018,0.0812033911017416,
4.));
#35810=CARTESIAN_POINT('Ctrl Pts',(-0.0967721750025885,0.0819369232370377,
4.));
#35811=CARTESIAN_POINT('Ctrl Pts',(-0.0959941513168557,0.0826601513985347,
4.));
#35812=CARTESIAN_POINT('Origin',(0.,0.,3.7));
#35813=CARTESIAN_POINT('Origin',(0.,0.,3.4));
#35814=CARTESIAN_POINT('Origin',(1.,0.,3.8));
#35815=CARTESIAN_POINT('',(0.8,2.44929359829471E-17,4.));
#35816=CARTESIAN_POINT('Origin',(1.,0.,4.));
#35817=CARTESIAN_POINT('',(0.8,2.44929359829471E-17,3.6));
#35818=CARTESIAN_POINT('',(0.8,2.44929359829471E-17,3.8));
#35819=CARTESIAN_POINT('Origin',(1.,0.,3.6));
#35820=CARTESIAN_POINT('Origin',(1.4,-0.6,3.6));
#35821=CARTESIAN_POINT('',(1.4,-0.6,3.6));
#35822=CARTESIAN_POINT('',(1.4,0.6,3.6));
#35823=CARTESIAN_POINT('',(1.4,-0.6,3.6));
#35824=CARTESIAN_POINT('',(1.4,0.6,4.));
#35825=CARTESIAN_POINT('',(1.4,0.6,3.6));
#35826=CARTESIAN_POINT('',(1.4,-0.6,4.));
#35827=CARTESIAN_POINT('',(1.4,-0.6,4.));
#35828=CARTESIAN_POINT('',(1.4,-0.6,3.6));
#35829=CARTESIAN_POINT('Origin',(0.7,0.,3.6));
#35830=CARTESIAN_POINT('',(0.4,0.6,3.6));
#35831=CARTESIAN_POINT('',(0.4,-0.6,3.6));
#35832=CARTESIAN_POINT('',(0.4,-0.3,3.6));
#35833=CARTESIAN_POINT('',(1.4,0.6,3.6));
#35834=CARTESIAN_POINT('',(0.,-0.6,3.6));
#35835=CARTESIAN_POINT('Origin',(0.4,0.6,2.6));
#35836=CARTESIAN_POINT('',(-0.4,0.6,4.));
#35837=CARTESIAN_POINT('',(0.4,0.6,4.));
#35838=CARTESIAN_POINT('',(0.4,0.6,2.6));
#35839=CARTESIAN_POINT('',(0.4,0.6,2.6));
#35840=CARTESIAN_POINT('',(-0.4,0.6,2.6));
#35841=CARTESIAN_POINT('',(0.4,0.6,2.6));
#35842=CARTESIAN_POINT('',(-0.4,0.6,2.6));
#35843=CARTESIAN_POINT('Origin',(0.4,-0.6,2.6));
#35844=CARTESIAN_POINT('',(0.4,-0.6,2.6));
#35845=CARTESIAN_POINT('',(0.4,-0.6,2.6));
#35846=CARTESIAN_POINT('',(0.4,-0.6,2.6));
#35847=CARTESIAN_POINT('Origin',(-0.4,-0.6,2.6));
#35848=CARTESIAN_POINT('',(-0.4,-0.6,4.));
#35849=CARTESIAN_POINT('',(-0.4,-0.6,4.));
#35850=CARTESIAN_POINT('',(-0.4,-0.6,2.6));
#35851=CARTESIAN_POINT('',(-0.4,-0.6,2.6));
#35852=CARTESIAN_POINT('',(-0.4,-0.6,2.6));
#35853=CARTESIAN_POINT('Origin',(-0.4,0.6,2.6));
#35854=CARTESIAN_POINT('',(-0.4,0.6,2.6));
#35855=CARTESIAN_POINT('',(-0.4,0.6,4.));
#35856=CARTESIAN_POINT('Origin',(0.,0.,4.));
#35857=CARTESIAN_POINT('Origin',(0.,0.,2.6));
#43952=UNCERTAINTY_MEASURE_WITH_UNIT(LENGTH_MEASURE(0.001),#43981,
'DISTANCE_ACCURACY_VALUE',
'Maximum model space distance between geometric entities at asserted c
onnectivities');
#43961=UNCERTAINTY_MEASURE_WITH_UNIT(LENGTH_MEASURE(0.001),#43981,
'DISTANCE_ACCURACY_VALUE',
'Maximum model space distance between geometric entities at asserted c
onnectivities');
#43971=(
GEOMETRIC_REPRESENTATION_CONTEXT(3)
GLOBAL_UNCERTAINTY_ASSIGNED_CONTEXT((#43952))
GLOBAL_UNIT_ASSIGNED_CONTEXT((#43981,#43983,#43984))
REPRESENTATION_CONTEXT('','3D')
);
#43980=(
GEOMETRIC_REPRESENTATION_CONTEXT(3)
GLOBAL_UNCERTAINTY_ASSIGNED_CONTEXT((#43961))
GLOBAL_UNIT_ASSIGNED_CONTEXT((#43981,#43983,#43984))
REPRESENTATION_CONTEXT('','3D')
);
#43981=(
LENGTH_UNIT()
NAMED_UNIT(*)
SI_UNIT(.CENTI.,.METRE.)
);
#43983=(
NAMED_UNIT(*)
PLANE_ANGLE_UNIT()
SI_UNIT($,.RADIAN.)
);
#43984=(
NAMED_UNIT(*)
SI_UNIT($,.STERADIAN.)
SOLID_ANGLE_UNIT()
);
#43994=SHAPE_DEFINITION_REPRESENTATION(#44012,#44064);
#44012=PRODUCT_DEFINITION_SHAPE('',$,#44083);
#44064=SHAPE_REPRESENTATION('',(#11983),#43971);
#44073=PRODUCT_DEFINITION_CONTEXT('part definition',#44129,'design');
#44083=PRODUCT_DEFINITION('Fixed contact terminal',
'Fixed contact terminal',#44101,#44073);
#44101=PRODUCT_DEFINITION_FORMATION('',$,#44140);
#44129=APPLICATION_CONTEXT(
'Core Data for Automotive Mechanical Design Process');
#44130=PRODUCT_CONTEXT('part definition',#44129,'mechanical');
#44140=PRODUCT('Fixed contact terminal','Fixed contact terminal',$,(#44130));
#44154=PRESENTATION_STYLE_ASSIGNMENT((#44166));
#44166=SURFACE_STYLE_USAGE(.BOTH.,#44178);
#44178=SURFACE_SIDE_STYLE('',(#44190));
#44190=SURFACE_STYLE_FILL_AREA(#44202);
#44202=FILL_AREA_STYLE('Contact gray',(#44214));
#44214=FILL_AREA_STYLE_COLOUR('Contact gray',#44226);
#44226=COLOUR_RGB('Contact gray',0.725490196078431,0.752941176470588,0.792156862745098);
ENDSEC;
END-ISO-10303-21;
